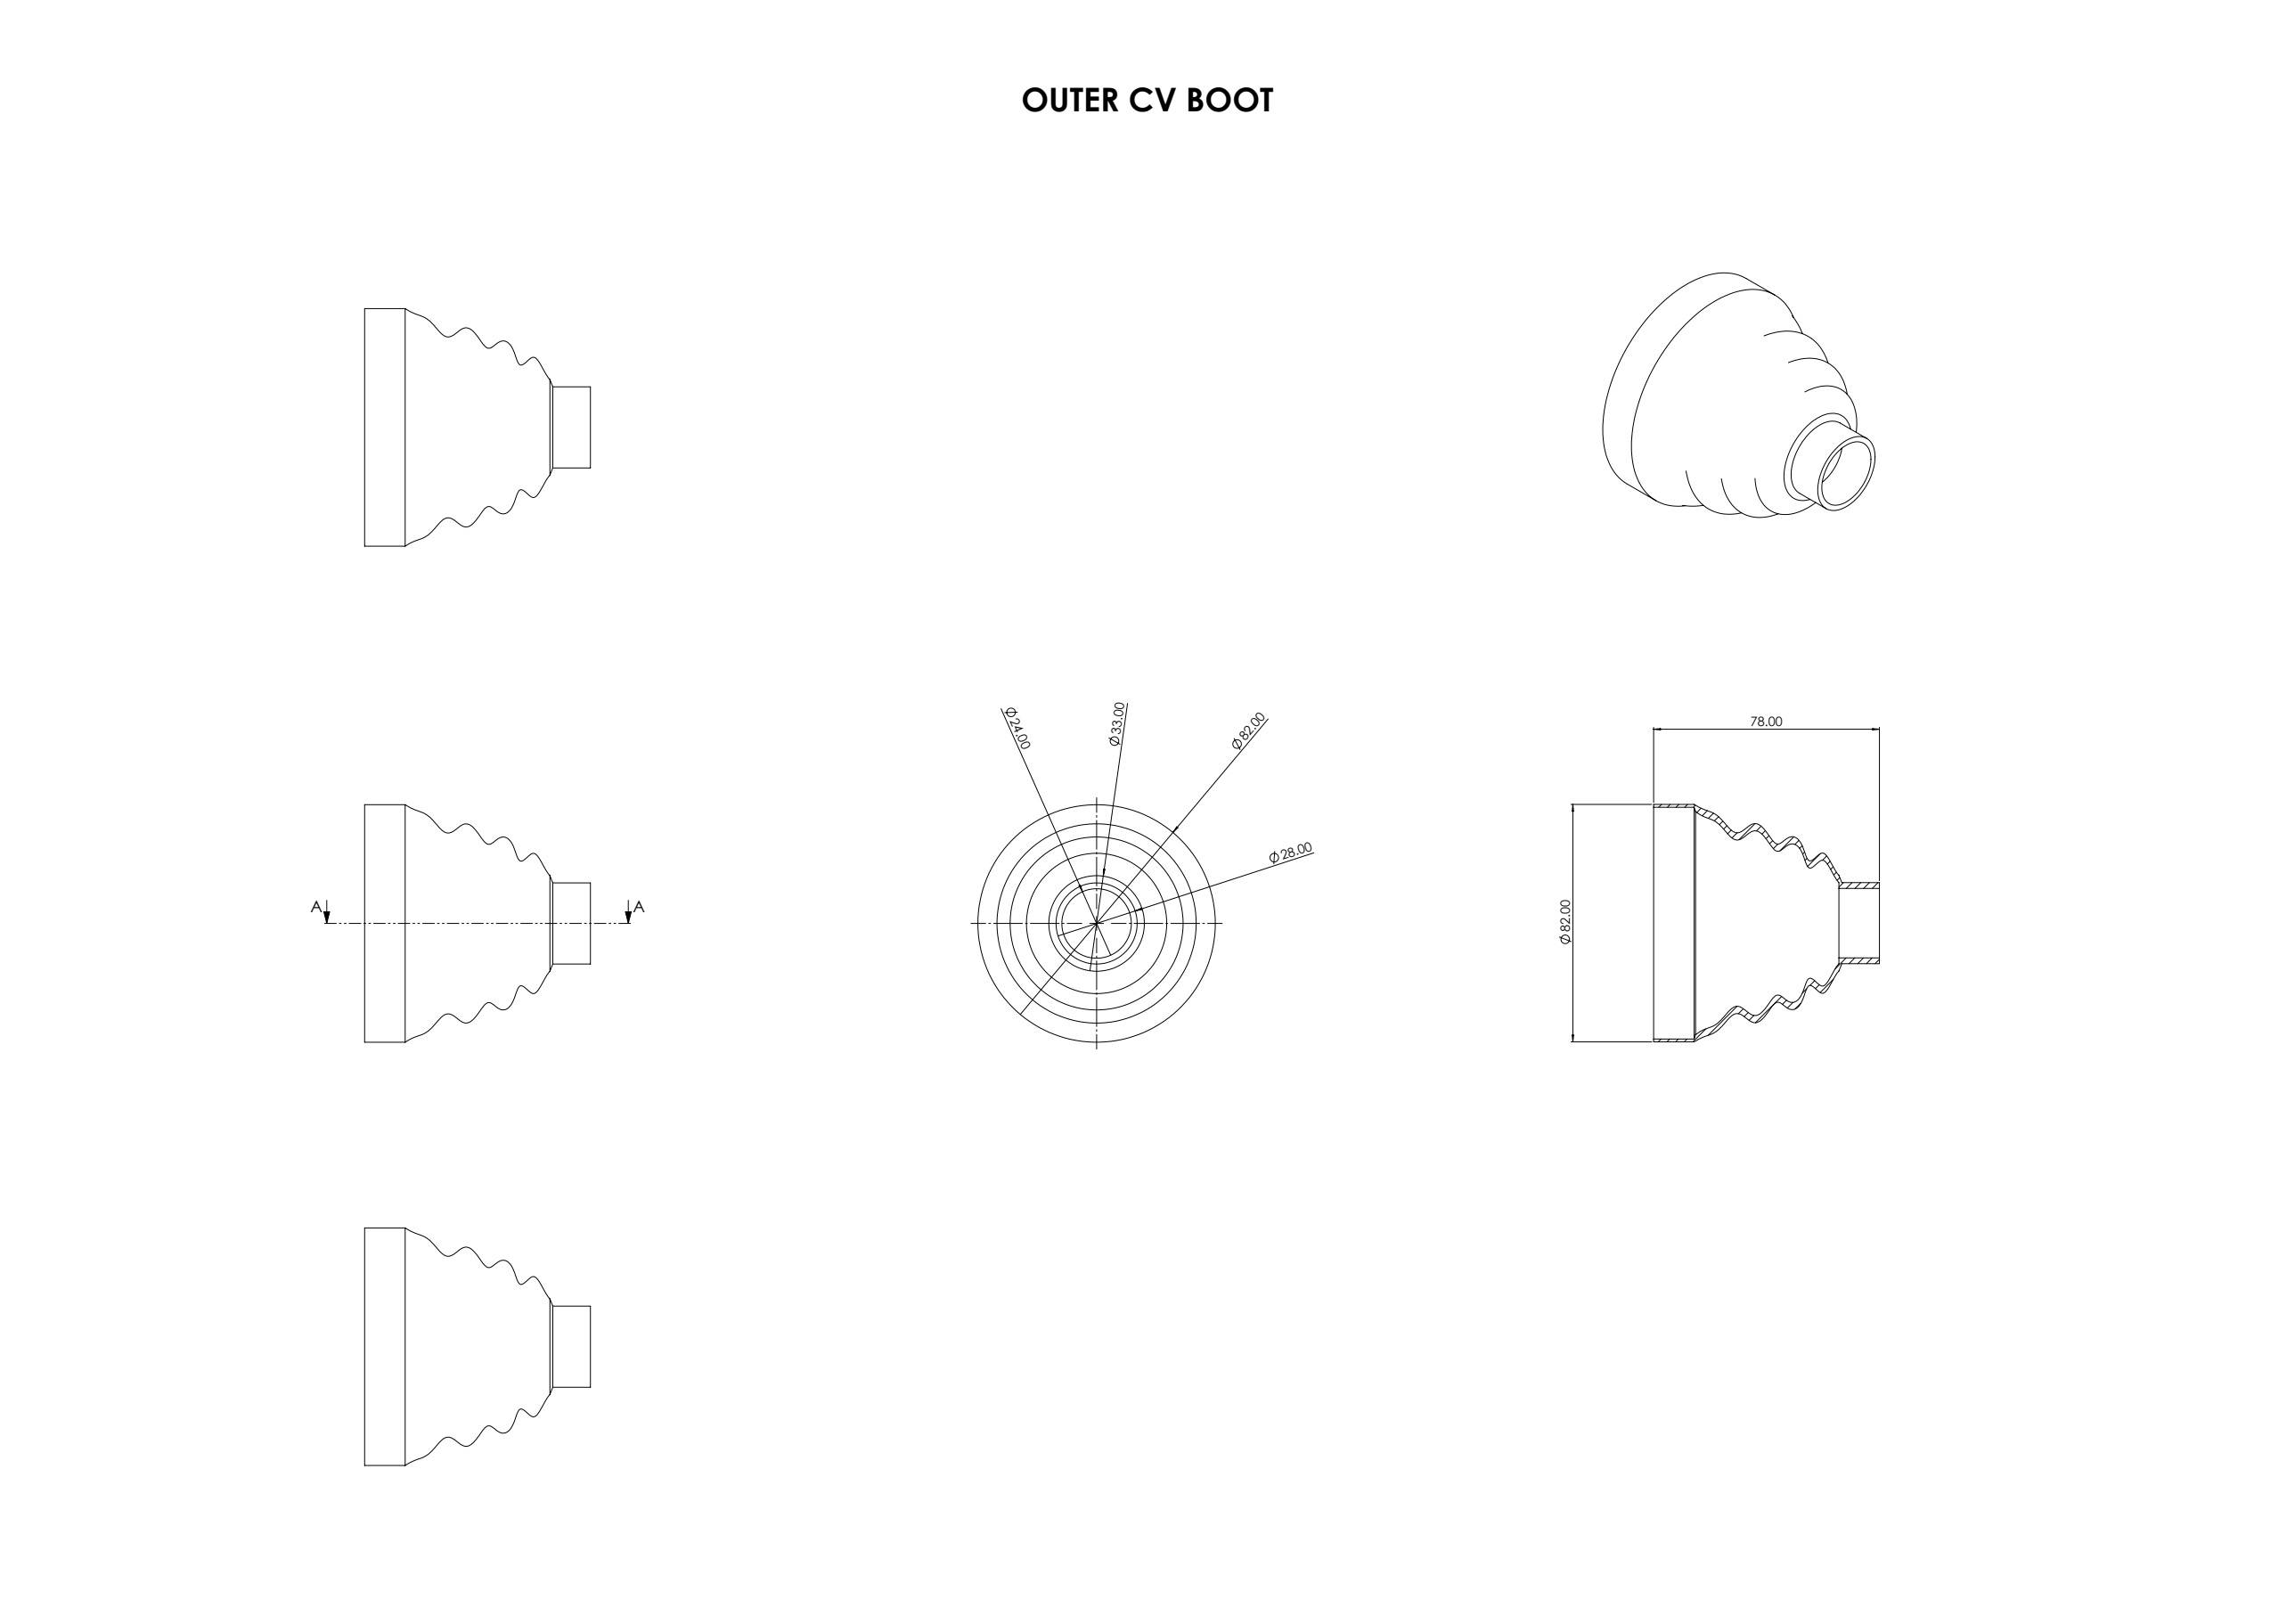
ISO-10303-21;
HEADER;
/* Generated by software containing ST-Developer
 * from STEP Tools, Inc. (www.steptools.com) 
 */

FILE_DESCRIPTION(
/* description */ (''),
/* implementation_level */ '2;1');

FILE_NAME(
/* name */ '07_Outer_CV_Boot.step',
/* time_stamp */ '2026-10-11T12:57:03-07:00',
/* author */ (''),
/* organization */ (''),
/* preprocessor_version */ 'ST-DEVELOPER v20.2',
/* originating_system */ 'Autodesk Translation Framework v15.15.0.0',
/* authorisation */ '');

FILE_SCHEMA (('AUTOMOTIVE_DESIGN { 1 0 10303 214 3 1 1 }'));
ENDSEC;

DATA;
#10=MECHANICAL_DESIGN_GEOMETRIC_PRESENTATION_REPRESENTATION('',(#262),#90374);
#228=SHAPE_REPRESENTATION_RELATIONSHIP('SRR','None',#90447,#245);
#245=ADVANCED_BREP_SHAPE_REPRESENTATION('',(#279),#90363);
#262=STYLED_ITEM('',(#90680),#279);
#279=MANIFOLD_SOLID_BREP('Body1',#40351);
#687=CONICAL_SURFACE('',#43806,15.25,1.19028994968254);
#688=CONICAL_SURFACE('',#43818,39.25,1.24904577239827);
#1066=FACE_BOUND('',#6231,.T.);
#1067=FACE_BOUND('',#6237,.T.);
#1068=FACE_BOUND('',#6240,.T.);
#1436=PLANE('',#43799);
#1437=PLANE('',#43810);
#1438=PLANE('',#43814);
#1831=(
BOUNDED_CURVE()
B_SPLINE_CURVE(5,(#82013,#82014,#82015,#82016,#82017,#82018,#82019,#82020,
#82021,#82022,#82023,#82024,#82025,#82026,#82027,#82028,#82029,#82030,#82031,
#82032,#82033,#82034,#82035,#82036,#82037,#82038,#82039,#82040,#82041,#82042,
#82043,#82044,#82045,#82046,#82047,#82048,#82049,#82050,#82051,#82052,#82053,
#82054,#82055,#82056,#82057,#82058,#82059,#82060,#82061,#82062,#82063,#82064,
#82065,#82066,#82067,#82068,#82069,#82070,#82071,#82072,#82073,#82074,#82075,
#82076,#82077,#82078,#82079,#82080,#82081,#82082,#82083,#82084,#82085,#82086,
#82087,#82088,#82089,#82090,#82091,#82092,#82093,#82094,#82095,#82096,#82097),
 .UNSPECIFIED.,.F.,.F.)
B_SPLINE_CURVE_WITH_KNOTS((6,1,1,1,1,1,1,1,1,1,1,1,1,1,1,1,1,1,1,1,1,1,
1,1,1,1,1,1,1,1,1,1,1,1,1,1,1,1,1,1,1,1,1,1,1,1,1,1,1,1,1,1,1,1,1,1,1,1,
1,1,1,1,1,1,1,1,1,1,1,1,1,1,1,1,1,1,1,1,1,1,6),(0.,0.0125,0.025,0.0375,
0.05,0.0625,0.075,0.0875,0.1,0.1125,0.125,0.1375,0.15,0.1625,0.175,0.1875,
0.2,0.2125,0.225,0.2375,0.25,0.2625,0.275,0.2875,0.3,0.3125,0.325,0.3375,
0.35,0.3625,0.375,0.3875,0.4,0.4125,0.425,0.4375,0.45,0.4625,0.475,0.4875,
0.5,0.5125,0.525,0.5375,0.55,0.5625,0.575,0.5875,0.6,0.6125,0.625,0.6375,
0.65,0.6625,0.675,0.6875,0.7,0.712499999999999,0.724999999999999,0.737499999999999,
0.749999999999999,0.762499999999999,0.774999999999999,0.787499999999999,
0.799999999999999,0.812499999999999,0.824999999999999,0.837499999999999,
0.849999999999999,0.862499999999999,0.874999999999999,0.887499999999999,
0.899999999999999,0.912499999999999,0.924999999999999,0.937499999999999,
0.949999999999999,0.962499999999999,0.974999999999999,0.987499999999998,
1.),.UNSPECIFIED.)
CURVE()
GEOMETRIC_REPRESENTATION_ITEM()
RATIONAL_B_SPLINE_CURVE((1.,1.,1.,1.,1.,1.,1.,1.,1.,1.,1.,1.,1.,1.,1.,1.,
1.,1.,1.,1.,1.,1.,1.,1.,1.,1.,1.,1.,1.,1.,1.,1.,1.,1.,1.,1.,1.,1.,1.,1.,
1.,1.,1.,1.,1.,1.,1.,1.,1.,1.,1.,1.,1.,1.,1.,1.,1.,1.,1.,1.,1.,1.,1.,1.,
1.,1.,1.,1.,1.,1.,1.,1.,1.,1.,1.,1.,1.,1.,1.,1.,1.,1.,1.,1.,1.))
REPRESENTATION_ITEM('')
);
#1832=(
BOUNDED_CURVE()
B_SPLINE_CURVE(5,(#82885,#82886,#82887,#82888,#82889,#82890,#82891,#82892,
#82893,#82894,#82895,#82896,#82897,#82898,#82899,#82900,#82901,#82902,#82903,
#82904,#82905,#82906,#82907,#82908,#82909,#82910,#82911,#82912,#82913,#82914,
#82915,#82916,#82917,#82918,#82919,#82920,#82921,#82922,#82923,#82924,#82925,
#82926,#82927,#82928,#82929,#82930,#82931,#82932,#82933,#82934,#82935,#82936,
#82937,#82938,#82939,#82940,#82941,#82942,#82943,#82944,#82945,#82946,#82947,
#82948,#82949,#82950,#82951,#82952,#82953,#82954,#82955,#82956,#82957,#82958,
#82959,#82960,#82961,#82962,#82963,#82964,#82965,#82966,#82967,#82968,#82969),
 .UNSPECIFIED.,.F.,.F.)
B_SPLINE_CURVE_WITH_KNOTS((6,1,1,1,1,1,1,1,1,1,1,1,1,1,1,1,1,1,1,1,1,1,
1,1,1,1,1,1,1,1,1,1,1,1,1,1,1,1,1,1,1,1,1,1,1,1,1,1,1,1,1,1,1,1,1,1,1,1,
1,1,1,1,1,1,1,1,1,1,1,1,1,1,1,1,1,1,1,1,1,1,6),(0.,0.0125,0.025,0.0375,
0.05,0.0625,0.075,0.0875,0.1,0.1125,0.125,0.1375,0.15,0.1625,0.175,0.1875,
0.2,0.2125,0.225,0.2375,0.25,0.2625,0.275,0.2875,0.3,0.3125,0.325,0.3375,
0.35,0.3625,0.375,0.3875,0.4,0.4125,0.425,0.4375,0.45,0.4625,0.475,0.4875,
0.5,0.5125,0.525,0.5375,0.55,0.5625,0.575,0.5875,0.6,0.6125,0.625,0.6375,
0.65,0.6625,0.675,0.6875,0.7,0.712499999999999,0.724999999999999,0.737499999999999,
0.749999999999999,0.762499999999999,0.774999999999999,0.787499999999999,
0.799999999999999,0.812499999999999,0.824999999999999,0.837499999999999,
0.849999999999999,0.862499999999999,0.874999999999999,0.887499999999999,
0.899999999999999,0.912499999999999,0.924999999999999,0.937499999999999,
0.949999999999999,0.962499999999999,0.974999999999999,0.987499999999998,
1.),.UNSPECIFIED.)
CURVE()
GEOMETRIC_REPRESENTATION_ITEM()
RATIONAL_B_SPLINE_CURVE((1.,1.,1.,1.,1.,1.,1.,1.,1.,1.,1.,1.,1.,1.,1.,1.,
1.,1.,1.,1.,1.,1.,1.,1.,1.,1.,1.,1.,1.,1.,1.,1.,1.,1.,1.,1.,1.,1.,1.,1.,
1.,1.,1.,1.,1.,1.,1.,1.,1.,1.,1.,1.,1.,1.,1.,1.,1.,1.,1.,1.,1.,1.,1.,1.,
1.,1.,1.,1.,1.,1.,1.,1.,1.,1.,1.,1.,1.,1.,1.,1.,1.,1.,1.,1.,1.))
REPRESENTATION_ITEM('')
);
#1934=(
BOUNDED_SURFACE()
B_SPLINE_SURFACE(5,2,((#81247,#81248,#81249,#81250,#81251,#81252,#81253,
#81254,#81255),(#81256,#81257,#81258,#81259,#81260,#81261,#81262,#81263,
#81264),(#81265,#81266,#81267,#81268,#81269,#81270,#81271,#81272,#81273),
(#81274,#81275,#81276,#81277,#81278,#81279,#81280,#81281,#81282),(#81283,
#81284,#81285,#81286,#81287,#81288,#81289,#81290,#81291),(#81292,#81293,
#81294,#81295,#81296,#81297,#81298,#81299,#81300),(#81301,#81302,#81303,
#81304,#81305,#81306,#81307,#81308,#81309),(#81310,#81311,#81312,#81313,
#81314,#81315,#81316,#81317,#81318),(#81319,#81320,#81321,#81322,#81323,
#81324,#81325,#81326,#81327),(#81328,#81329,#81330,#81331,#81332,#81333,
#81334,#81335,#81336),(#81337,#81338,#81339,#81340,#81341,#81342,#81343,
#81344,#81345),(#81346,#81347,#81348,#81349,#81350,#81351,#81352,#81353,
#81354),(#81355,#81356,#81357,#81358,#81359,#81360,#81361,#81362,#81363),
(#81364,#81365,#81366,#81367,#81368,#81369,#81370,#81371,#81372),(#81373,
#81374,#81375,#81376,#81377,#81378,#81379,#81380,#81381),(#81382,#81383,
#81384,#81385,#81386,#81387,#81388,#81389,#81390),(#81391,#81392,#81393,
#81394,#81395,#81396,#81397,#81398,#81399),(#81400,#81401,#81402,#81403,
#81404,#81405,#81406,#81407,#81408),(#81409,#81410,#81411,#81412,#81413,
#81414,#81415,#81416,#81417),(#81418,#81419,#81420,#81421,#81422,#81423,
#81424,#81425,#81426),(#81427,#81428,#81429,#81430,#81431,#81432,#81433,
#81434,#81435),(#81436,#81437,#81438,#81439,#81440,#81441,#81442,#81443,
#81444),(#81445,#81446,#81447,#81448,#81449,#81450,#81451,#81452,#81453),
(#81454,#81455,#81456,#81457,#81458,#81459,#81460,#81461,#81462),(#81463,
#81464,#81465,#81466,#81467,#81468,#81469,#81470,#81471),(#81472,#81473,
#81474,#81475,#81476,#81477,#81478,#81479,#81480),(#81481,#81482,#81483,
#81484,#81485,#81486,#81487,#81488,#81489),(#81490,#81491,#81492,#81493,
#81494,#81495,#81496,#81497,#81498),(#81499,#81500,#81501,#81502,#81503,
#81504,#81505,#81506,#81507),(#81508,#81509,#81510,#81511,#81512,#81513,
#81514,#81515,#81516),(#81517,#81518,#81519,#81520,#81521,#81522,#81523,
#81524,#81525),(#81526,#81527,#81528,#81529,#81530,#81531,#81532,#81533,
#81534),(#81535,#81536,#81537,#81538,#81539,#81540,#81541,#81542,#81543),
(#81544,#81545,#81546,#81547,#81548,#81549,#81550,#81551,#81552),(#81553,
#81554,#81555,#81556,#81557,#81558,#81559,#81560,#81561),(#81562,#81563,
#81564,#81565,#81566,#81567,#81568,#81569,#81570),(#81571,#81572,#81573,
#81574,#81575,#81576,#81577,#81578,#81579),(#81580,#81581,#81582,#81583,
#81584,#81585,#81586,#81587,#81588),(#81589,#81590,#81591,#81592,#81593,
#81594,#81595,#81596,#81597),(#81598,#81599,#81600,#81601,#81602,#81603,
#81604,#81605,#81606),(#81607,#81608,#81609,#81610,#81611,#81612,#81613,
#81614,#81615),(#81616,#81617,#81618,#81619,#81620,#81621,#81622,#81623,
#81624),(#81625,#81626,#81627,#81628,#81629,#81630,#81631,#81632,#81633),
(#81634,#81635,#81636,#81637,#81638,#81639,#81640,#81641,#81642),(#81643,
#81644,#81645,#81646,#81647,#81648,#81649,#81650,#81651),(#81652,#81653,
#81654,#81655,#81656,#81657,#81658,#81659,#81660),(#81661,#81662,#81663,
#81664,#81665,#81666,#81667,#81668,#81669),(#81670,#81671,#81672,#81673,
#81674,#81675,#81676,#81677,#81678),(#81679,#81680,#81681,#81682,#81683,
#81684,#81685,#81686,#81687),(#81688,#81689,#81690,#81691,#81692,#81693,
#81694,#81695,#81696),(#81697,#81698,#81699,#81700,#81701,#81702,#81703,
#81704,#81705),(#81706,#81707,#81708,#81709,#81710,#81711,#81712,#81713,
#81714),(#81715,#81716,#81717,#81718,#81719,#81720,#81721,#81722,#81723),
(#81724,#81725,#81726,#81727,#81728,#81729,#81730,#81731,#81732),(#81733,
#81734,#81735,#81736,#81737,#81738,#81739,#81740,#81741),(#81742,#81743,
#81744,#81745,#81746,#81747,#81748,#81749,#81750),(#81751,#81752,#81753,
#81754,#81755,#81756,#81757,#81758,#81759),(#81760,#81761,#81762,#81763,
#81764,#81765,#81766,#81767,#81768),(#81769,#81770,#81771,#81772,#81773,
#81774,#81775,#81776,#81777),(#81778,#81779,#81780,#81781,#81782,#81783,
#81784,#81785,#81786),(#81787,#81788,#81789,#81790,#81791,#81792,#81793,
#81794,#81795),(#81796,#81797,#81798,#81799,#81800,#81801,#81802,#81803,
#81804),(#81805,#81806,#81807,#81808,#81809,#81810,#81811,#81812,#81813),
(#81814,#81815,#81816,#81817,#81818,#81819,#81820,#81821,#81822),(#81823,
#81824,#81825,#81826,#81827,#81828,#81829,#81830,#81831),(#81832,#81833,
#81834,#81835,#81836,#81837,#81838,#81839,#81840),(#81841,#81842,#81843,
#81844,#81845,#81846,#81847,#81848,#81849),(#81850,#81851,#81852,#81853,
#81854,#81855,#81856,#81857,#81858),(#81859,#81860,#81861,#81862,#81863,
#81864,#81865,#81866,#81867),(#81868,#81869,#81870,#81871,#81872,#81873,
#81874,#81875,#81876),(#81877,#81878,#81879,#81880,#81881,#81882,#81883,
#81884,#81885),(#81886,#81887,#81888,#81889,#81890,#81891,#81892,#81893,
#81894),(#81895,#81896,#81897,#81898,#81899,#81900,#81901,#81902,#81903),
(#81904,#81905,#81906,#81907,#81908,#81909,#81910,#81911,#81912),(#81913,
#81914,#81915,#81916,#81917,#81918,#81919,#81920,#81921),(#81922,#81923,
#81924,#81925,#81926,#81927,#81928,#81929,#81930),(#81931,#81932,#81933,
#81934,#81935,#81936,#81937,#81938,#81939),(#81940,#81941,#81942,#81943,
#81944,#81945,#81946,#81947,#81948),(#81949,#81950,#81951,#81952,#81953,
#81954,#81955,#81956,#81957),(#81958,#81959,#81960,#81961,#81962,#81963,
#81964,#81965,#81966),(#81967,#81968,#81969,#81970,#81971,#81972,#81973,
#81974,#81975),(#81976,#81977,#81978,#81979,#81980,#81981,#81982,#81983,
#81984),(#81985,#81986,#81987,#81988,#81989,#81990,#81991,#81992,#81993),
(#81994,#81995,#81996,#81997,#81998,#81999,#82000,#82001,#82002),(#82003,
#82004,#82005,#82006,#82007,#82008,#82009,#82010,#82011)),.UNSPECIFIED.,
 .F.,.T.,.F.)
B_SPLINE_SURFACE_WITH_KNOTS((6,1,1,1,1,1,1,1,1,1,1,1,1,1,1,1,1,1,1,1,1,
1,1,1,1,1,1,1,1,1,1,1,1,1,1,1,1,1,1,1,1,1,1,1,1,1,1,1,1,1,1,1,1,1,1,1,1,
1,1,1,1,1,1,1,1,1,1,1,1,1,1,1,1,1,1,1,1,1,1,1,6),(3,2,2,2,3),(-1.,-0.987499999999998,
-0.974999999999999,-0.962499999999999,-0.949999999999999,-0.937499999999999,
-0.924999999999999,-0.912499999999999,-0.899999999999999,-0.887499999999999,
-0.874999999999999,-0.862499999999999,-0.849999999999999,-0.837499999999999,
-0.824999999999999,-0.812499999999999,-0.799999999999999,-0.787499999999999,
-0.774999999999999,-0.762499999999999,-0.749999999999999,-0.737499999999999,
-0.724999999999999,-0.712499999999999,-0.7,-0.6875,-0.675,-0.6625,-0.65,
-0.6375,-0.625,-0.6125,-0.6,-0.5875,-0.575,-0.5625,-0.55,-0.5375,-0.525,
-0.5125,-0.5,-0.4875,-0.475,-0.4625,-0.45,-0.4375,-0.425,-0.4125,-0.4,-0.3875,
-0.375,-0.3625,-0.35,-0.3375,-0.325,-0.3125,-0.3,-0.2875,-0.275,-0.2625,
-0.25,-0.2375,-0.225,-0.2125,-0.2,-0.1875,-0.175,-0.1625,-0.15,-0.1375,
-0.125,-0.1125,-0.1,-0.0875,-0.075,-0.0625,-0.05,-0.0375,-0.025,-0.0125,
0.),(0.,1.5707963267949,3.14159265358979,4.71238898038469,6.28318530717959),
 .UNSPECIFIED.)
GEOMETRIC_REPRESENTATION_ITEM()
RATIONAL_B_SPLINE_SURFACE(((1.,0.707106781186548,1.,0.707106781186548,1.,
0.707106781186548,1.,0.707106781186548,1.),(1.,0.707106781186548,1.,0.707106781186548,
1.,0.707106781186548,1.,0.707106781186548,1.),(1.,0.707106781186548,1.,
0.707106781186548,1.,0.707106781186548,1.,0.707106781186548,1.),(1.,0.707106781186548,
1.,0.707106781186548,1.,0.707106781186548,1.,0.707106781186548,1.),(1.,
0.707106781186548,1.,0.707106781186548,1.,0.707106781186548,1.,0.707106781186548,
1.),(1.,0.707106781186548,1.,0.707106781186548,1.,0.707106781186548,1.,
0.707106781186548,1.),(1.,0.707106781186548,1.,0.707106781186548,1.,0.707106781186548,
1.,0.707106781186548,1.),(1.,0.707106781186548,1.,0.707106781186548,1.,
0.707106781186548,1.,0.707106781186548,1.),(1.,0.707106781186548,1.,0.707106781186548,
1.,0.707106781186548,1.,0.707106781186548,1.),(1.,0.707106781186548,1.,
0.707106781186548,1.,0.707106781186548,1.,0.707106781186548,1.),(1.,0.707106781186548,
1.,0.707106781186548,1.,0.707106781186548,1.,0.707106781186548,1.),(1.,
0.707106781186548,1.,0.707106781186548,1.,0.707106781186548,1.,0.707106781186548,
1.),(1.,0.707106781186548,1.,0.707106781186548,1.,0.707106781186548,1.,
0.707106781186548,1.),(1.,0.707106781186548,1.,0.707106781186548,1.,0.707106781186548,
1.,0.707106781186548,1.),(1.,0.707106781186548,1.,0.707106781186548,1.,
0.707106781186548,1.,0.707106781186548,1.),(1.,0.707106781186548,1.,0.707106781186548,
1.,0.707106781186548,1.,0.707106781186548,1.),(1.,0.707106781186548,1.,
0.707106781186548,1.,0.707106781186548,1.,0.707106781186548,1.),(1.,0.707106781186548,
1.,0.707106781186548,1.,0.707106781186548,1.,0.707106781186548,1.),(1.,
0.707106781186548,1.,0.707106781186548,1.,0.707106781186548,1.,0.707106781186548,
1.),(1.,0.707106781186548,1.,0.707106781186548,1.,0.707106781186548,1.,
0.707106781186548,1.),(1.,0.707106781186548,1.,0.707106781186548,1.,0.707106781186548,
1.,0.707106781186548,1.),(1.,0.707106781186548,1.,0.707106781186548,1.,
0.707106781186548,1.,0.707106781186548,1.),(1.,0.707106781186548,1.,0.707106781186548,
1.,0.707106781186548,1.,0.707106781186548,1.),(1.,0.707106781186548,1.,
0.707106781186548,1.,0.707106781186548,1.,0.707106781186548,1.),(1.,0.707106781186548,
1.,0.707106781186548,1.,0.707106781186548,1.,0.707106781186548,1.),(1.,
0.707106781186548,1.,0.707106781186548,1.,0.707106781186548,1.,0.707106781186548,
1.),(1.,0.707106781186548,1.,0.707106781186548,1.,0.707106781186548,1.,
0.707106781186548,1.),(1.,0.707106781186548,1.,0.707106781186548,1.,0.707106781186548,
1.,0.707106781186548,1.),(1.,0.707106781186548,1.,0.707106781186548,1.,
0.707106781186548,1.,0.707106781186548,1.),(1.,0.707106781186548,1.,0.707106781186548,
1.,0.707106781186548,1.,0.707106781186548,1.),(1.,0.707106781186548,1.,
0.707106781186548,1.,0.707106781186548,1.,0.707106781186548,1.),(1.,0.707106781186548,
1.,0.707106781186548,1.,0.707106781186548,1.,0.707106781186548,1.),(1.,
0.707106781186548,1.,0.707106781186548,1.,0.707106781186548,1.,0.707106781186548,
1.),(1.,0.707106781186548,1.,0.707106781186548,1.,0.707106781186548,1.,
0.707106781186548,1.),(1.,0.707106781186548,1.,0.707106781186548,1.,0.707106781186548,
1.,0.707106781186548,1.),(1.,0.707106781186548,1.,0.707106781186548,1.,
0.707106781186548,1.,0.707106781186548,1.),(1.,0.707106781186548,1.,0.707106781186548,
1.,0.707106781186548,1.,0.707106781186548,1.),(1.,0.707106781186548,1.,
0.707106781186548,1.,0.707106781186548,1.,0.707106781186548,1.),(1.,0.707106781186548,
1.,0.707106781186548,1.,0.707106781186548,1.,0.707106781186548,1.),(1.,
0.707106781186548,1.,0.707106781186548,1.,0.707106781186548,1.,0.707106781186548,
1.),(1.,0.707106781186548,1.,0.707106781186548,1.,0.707106781186548,1.,
0.707106781186548,1.),(1.,0.707106781186548,1.,0.707106781186548,1.,0.707106781186548,
1.,0.707106781186548,1.),(1.,0.707106781186548,1.,0.707106781186548,1.,
0.707106781186548,1.,0.707106781186548,1.),(1.,0.707106781186548,1.,0.707106781186548,
1.,0.707106781186548,1.,0.707106781186548,1.),(1.,0.707106781186548,1.,
0.707106781186548,1.,0.707106781186548,1.,0.707106781186548,1.),(1.,0.707106781186548,
1.,0.707106781186548,1.,0.707106781186548,1.,0.707106781186548,1.),(1.,
0.707106781186548,1.,0.707106781186548,1.,0.707106781186548,1.,0.707106781186548,
1.),(1.,0.707106781186548,1.,0.707106781186548,1.,0.707106781186548,1.,
0.707106781186548,1.),(1.,0.707106781186548,1.,0.707106781186548,1.,0.707106781186548,
1.,0.707106781186548,1.),(1.,0.707106781186548,1.,0.707106781186548,1.,
0.707106781186548,1.,0.707106781186548,1.),(1.,0.707106781186548,1.,0.707106781186548,
1.,0.707106781186548,1.,0.707106781186548,1.),(1.,0.707106781186548,1.,
0.707106781186548,1.,0.707106781186548,1.,0.707106781186548,1.),(1.,0.707106781186548,
1.,0.707106781186548,1.,0.707106781186548,1.,0.707106781186548,1.),(1.,
0.707106781186548,1.,0.707106781186548,1.,0.707106781186548,1.,0.707106781186548,
1.),(1.,0.707106781186548,1.,0.707106781186548,1.,0.707106781186548,1.,
0.707106781186548,1.),(1.,0.707106781186548,1.,0.707106781186548,1.,0.707106781186548,
1.,0.707106781186548,1.),(1.,0.707106781186548,1.,0.707106781186548,1.,
0.707106781186548,1.,0.707106781186548,1.),(1.,0.707106781186548,1.,0.707106781186548,
1.,0.707106781186548,1.,0.707106781186548,1.),(1.,0.707106781186548,1.,
0.707106781186548,1.,0.707106781186548,1.,0.707106781186548,1.),(1.,0.707106781186548,
1.,0.707106781186548,1.,0.707106781186548,1.,0.707106781186548,1.),(1.,
0.707106781186548,1.,0.707106781186548,1.,0.707106781186548,1.,0.707106781186548,
1.),(1.,0.707106781186548,1.,0.707106781186548,1.,0.707106781186548,1.,
0.707106781186548,1.),(1.,0.707106781186548,1.,0.707106781186548,1.,0.707106781186548,
1.,0.707106781186548,1.),(1.,0.707106781186548,1.,0.707106781186548,1.,
0.707106781186548,1.,0.707106781186548,1.),(1.,0.707106781186548,1.,0.707106781186548,
1.,0.707106781186548,1.,0.707106781186548,1.),(1.,0.707106781186548,1.,
0.707106781186548,1.,0.707106781186548,1.,0.707106781186548,1.),(1.,0.707106781186548,
1.,0.707106781186548,1.,0.707106781186548,1.,0.707106781186548,1.),(1.,
0.707106781186548,1.,0.707106781186548,1.,0.707106781186548,1.,0.707106781186548,
1.),(1.,0.707106781186548,1.,0.707106781186548,1.,0.707106781186548,1.,
0.707106781186548,1.),(1.,0.707106781186548,1.,0.707106781186548,1.,0.707106781186548,
1.,0.707106781186548,1.),(1.,0.707106781186548,1.,0.707106781186548,1.,
0.707106781186548,1.,0.707106781186548,1.),(1.,0.707106781186548,1.,0.707106781186548,
1.,0.707106781186548,1.,0.707106781186548,1.),(1.,0.707106781186548,1.,
0.707106781186548,1.,0.707106781186548,1.,0.707106781186548,1.),(1.,0.707106781186548,
1.,0.707106781186548,1.,0.707106781186548,1.,0.707106781186548,1.),(1.,
0.707106781186548,1.,0.707106781186548,1.,0.707106781186548,1.,0.707106781186548,
1.),(1.,0.707106781186548,1.,0.707106781186548,1.,0.707106781186548,1.,
0.707106781186548,1.),(1.,0.707106781186548,1.,0.707106781186548,1.,0.707106781186548,
1.,0.707106781186548,1.),(1.,0.707106781186548,1.,0.707106781186548,1.,
0.707106781186548,1.,0.707106781186548,1.),(1.,0.707106781186548,1.,0.707106781186548,
1.,0.707106781186548,1.,0.707106781186548,1.),(1.,0.707106781186548,1.,
0.707106781186548,1.,0.707106781186548,1.,0.707106781186548,1.),(1.,0.707106781186548,
1.,0.707106781186548,1.,0.707106781186548,1.,0.707106781186548,1.),(1.,
0.707106781186548,1.,0.707106781186548,1.,0.707106781186548,1.,0.707106781186548,
1.),(1.,0.707106781186548,1.,0.707106781186548,1.,0.707106781186548,1.,
0.707106781186548,1.),(1.,0.707106781186548,1.,0.707106781186548,1.,0.707106781186548,
1.,0.707106781186548,1.),(1.,0.707106781186548,1.,0.707106781186548,1.,
0.707106781186548,1.,0.707106781186548,1.)))
REPRESENTATION_ITEM('')
SURFACE()
);
#1935=(
BOUNDED_SURFACE()
B_SPLINE_SURFACE(5,2,((#82119,#82120,#82121,#82122,#82123,#82124,#82125,
#82126,#82127),(#82128,#82129,#82130,#82131,#82132,#82133,#82134,#82135,
#82136),(#82137,#82138,#82139,#82140,#82141,#82142,#82143,#82144,#82145),
(#82146,#82147,#82148,#82149,#82150,#82151,#82152,#82153,#82154),(#82155,
#82156,#82157,#82158,#82159,#82160,#82161,#82162,#82163),(#82164,#82165,
#82166,#82167,#82168,#82169,#82170,#82171,#82172),(#82173,#82174,#82175,
#82176,#82177,#82178,#82179,#82180,#82181),(#82182,#82183,#82184,#82185,
#82186,#82187,#82188,#82189,#82190),(#82191,#82192,#82193,#82194,#82195,
#82196,#82197,#82198,#82199),(#82200,#82201,#82202,#82203,#82204,#82205,
#82206,#82207,#82208),(#82209,#82210,#82211,#82212,#82213,#82214,#82215,
#82216,#82217),(#82218,#82219,#82220,#82221,#82222,#82223,#82224,#82225,
#82226),(#82227,#82228,#82229,#82230,#82231,#82232,#82233,#82234,#82235),
(#82236,#82237,#82238,#82239,#82240,#82241,#82242,#82243,#82244),(#82245,
#82246,#82247,#82248,#82249,#82250,#82251,#82252,#82253),(#82254,#82255,
#82256,#82257,#82258,#82259,#82260,#82261,#82262),(#82263,#82264,#82265,
#82266,#82267,#82268,#82269,#82270,#82271),(#82272,#82273,#82274,#82275,
#82276,#82277,#82278,#82279,#82280),(#82281,#82282,#82283,#82284,#82285,
#82286,#82287,#82288,#82289),(#82290,#82291,#82292,#82293,#82294,#82295,
#82296,#82297,#82298),(#82299,#82300,#82301,#82302,#82303,#82304,#82305,
#82306,#82307),(#82308,#82309,#82310,#82311,#82312,#82313,#82314,#82315,
#82316),(#82317,#82318,#82319,#82320,#82321,#82322,#82323,#82324,#82325),
(#82326,#82327,#82328,#82329,#82330,#82331,#82332,#82333,#82334),(#82335,
#82336,#82337,#82338,#82339,#82340,#82341,#82342,#82343),(#82344,#82345,
#82346,#82347,#82348,#82349,#82350,#82351,#82352),(#82353,#82354,#82355,
#82356,#82357,#82358,#82359,#82360,#82361),(#82362,#82363,#82364,#82365,
#82366,#82367,#82368,#82369,#82370),(#82371,#82372,#82373,#82374,#82375,
#82376,#82377,#82378,#82379),(#82380,#82381,#82382,#82383,#82384,#82385,
#82386,#82387,#82388),(#82389,#82390,#82391,#82392,#82393,#82394,#82395,
#82396,#82397),(#82398,#82399,#82400,#82401,#82402,#82403,#82404,#82405,
#82406),(#82407,#82408,#82409,#82410,#82411,#82412,#82413,#82414,#82415),
(#82416,#82417,#82418,#82419,#82420,#82421,#82422,#82423,#82424),(#82425,
#82426,#82427,#82428,#82429,#82430,#82431,#82432,#82433),(#82434,#82435,
#82436,#82437,#82438,#82439,#82440,#82441,#82442),(#82443,#82444,#82445,
#82446,#82447,#82448,#82449,#82450,#82451),(#82452,#82453,#82454,#82455,
#82456,#82457,#82458,#82459,#82460),(#82461,#82462,#82463,#82464,#82465,
#82466,#82467,#82468,#82469),(#82470,#82471,#82472,#82473,#82474,#82475,
#82476,#82477,#82478),(#82479,#82480,#82481,#82482,#82483,#82484,#82485,
#82486,#82487),(#82488,#82489,#82490,#82491,#82492,#82493,#82494,#82495,
#82496),(#82497,#82498,#82499,#82500,#82501,#82502,#82503,#82504,#82505),
(#82506,#82507,#82508,#82509,#82510,#82511,#82512,#82513,#82514),(#82515,
#82516,#82517,#82518,#82519,#82520,#82521,#82522,#82523),(#82524,#82525,
#82526,#82527,#82528,#82529,#82530,#82531,#82532),(#82533,#82534,#82535,
#82536,#82537,#82538,#82539,#82540,#82541),(#82542,#82543,#82544,#82545,
#82546,#82547,#82548,#82549,#82550),(#82551,#82552,#82553,#82554,#82555,
#82556,#82557,#82558,#82559),(#82560,#82561,#82562,#82563,#82564,#82565,
#82566,#82567,#82568),(#82569,#82570,#82571,#82572,#82573,#82574,#82575,
#82576,#82577),(#82578,#82579,#82580,#82581,#82582,#82583,#82584,#82585,
#82586),(#82587,#82588,#82589,#82590,#82591,#82592,#82593,#82594,#82595),
(#82596,#82597,#82598,#82599,#82600,#82601,#82602,#82603,#82604),(#82605,
#82606,#82607,#82608,#82609,#82610,#82611,#82612,#82613),(#82614,#82615,
#82616,#82617,#82618,#82619,#82620,#82621,#82622),(#82623,#82624,#82625,
#82626,#82627,#82628,#82629,#82630,#82631),(#82632,#82633,#82634,#82635,
#82636,#82637,#82638,#82639,#82640),(#82641,#82642,#82643,#82644,#82645,
#82646,#82647,#82648,#82649),(#82650,#82651,#82652,#82653,#82654,#82655,
#82656,#82657,#82658),(#82659,#82660,#82661,#82662,#82663,#82664,#82665,
#82666,#82667),(#82668,#82669,#82670,#82671,#82672,#82673,#82674,#82675,
#82676),(#82677,#82678,#82679,#82680,#82681,#82682,#82683,#82684,#82685),
(#82686,#82687,#82688,#82689,#82690,#82691,#82692,#82693,#82694),(#82695,
#82696,#82697,#82698,#82699,#82700,#82701,#82702,#82703),(#82704,#82705,
#82706,#82707,#82708,#82709,#82710,#82711,#82712),(#82713,#82714,#82715,
#82716,#82717,#82718,#82719,#82720,#82721),(#82722,#82723,#82724,#82725,
#82726,#82727,#82728,#82729,#82730),(#82731,#82732,#82733,#82734,#82735,
#82736,#82737,#82738,#82739),(#82740,#82741,#82742,#82743,#82744,#82745,
#82746,#82747,#82748),(#82749,#82750,#82751,#82752,#82753,#82754,#82755,
#82756,#82757),(#82758,#82759,#82760,#82761,#82762,#82763,#82764,#82765,
#82766),(#82767,#82768,#82769,#82770,#82771,#82772,#82773,#82774,#82775),
(#82776,#82777,#82778,#82779,#82780,#82781,#82782,#82783,#82784),(#82785,
#82786,#82787,#82788,#82789,#82790,#82791,#82792,#82793),(#82794,#82795,
#82796,#82797,#82798,#82799,#82800,#82801,#82802),(#82803,#82804,#82805,
#82806,#82807,#82808,#82809,#82810,#82811),(#82812,#82813,#82814,#82815,
#82816,#82817,#82818,#82819,#82820),(#82821,#82822,#82823,#82824,#82825,
#82826,#82827,#82828,#82829),(#82830,#82831,#82832,#82833,#82834,#82835,
#82836,#82837,#82838),(#82839,#82840,#82841,#82842,#82843,#82844,#82845,
#82846,#82847),(#82848,#82849,#82850,#82851,#82852,#82853,#82854,#82855,
#82856),(#82857,#82858,#82859,#82860,#82861,#82862,#82863,#82864,#82865),
(#82866,#82867,#82868,#82869,#82870,#82871,#82872,#82873,#82874),(#82875,
#82876,#82877,#82878,#82879,#82880,#82881,#82882,#82883)),.UNSPECIFIED.,
 .F.,.T.,.F.)
B_SPLINE_SURFACE_WITH_KNOTS((6,1,1,1,1,1,1,1,1,1,1,1,1,1,1,1,1,1,1,1,1,
1,1,1,1,1,1,1,1,1,1,1,1,1,1,1,1,1,1,1,1,1,1,1,1,1,1,1,1,1,1,1,1,1,1,1,1,
1,1,1,1,1,1,1,1,1,1,1,1,1,1,1,1,1,1,1,1,1,1,1,6),(3,2,2,2,3),(-1.,-0.987499999999998,
-0.974999999999999,-0.962499999999999,-0.949999999999999,-0.937499999999999,
-0.924999999999999,-0.912499999999999,-0.899999999999999,-0.887499999999999,
-0.874999999999999,-0.862499999999999,-0.849999999999999,-0.837499999999999,
-0.824999999999999,-0.812499999999999,-0.799999999999999,-0.787499999999999,
-0.774999999999999,-0.762499999999999,-0.749999999999999,-0.737499999999999,
-0.724999999999999,-0.712499999999999,-0.7,-0.6875,-0.675,-0.6625,-0.65,
-0.6375,-0.625,-0.6125,-0.6,-0.5875,-0.575,-0.5625,-0.55,-0.5375,-0.525,
-0.5125,-0.5,-0.4875,-0.475,-0.4625,-0.45,-0.4375,-0.425,-0.4125,-0.4,-0.3875,
-0.375,-0.3625,-0.35,-0.3375,-0.325,-0.3125,-0.3,-0.2875,-0.275,-0.2625,
-0.25,-0.2375,-0.225,-0.2125,-0.2,-0.1875,-0.175,-0.1625,-0.15,-0.1375,
-0.125,-0.1125,-0.1,-0.0875,-0.075,-0.0625,-0.05,-0.0375,-0.025,-0.0125,
0.),(0.,1.5707963267949,3.14159265358979,4.71238898038469,6.28318530717959),
 .UNSPECIFIED.)
GEOMETRIC_REPRESENTATION_ITEM()
RATIONAL_B_SPLINE_SURFACE(((1.,0.707106781186548,1.,0.707106781186548,1.,
0.707106781186548,1.,0.707106781186548,1.),(1.,0.707106781186548,1.,0.707106781186548,
1.,0.707106781186548,1.,0.707106781186548,1.),(1.,0.707106781186548,1.,
0.707106781186548,1.,0.707106781186548,1.,0.707106781186548,1.),(1.,0.707106781186548,
1.,0.707106781186548,1.,0.707106781186548,1.,0.707106781186548,1.),(1.,
0.707106781186548,1.,0.707106781186548,1.,0.707106781186548,1.,0.707106781186548,
1.),(1.,0.707106781186548,1.,0.707106781186548,1.,0.707106781186548,1.,
0.707106781186548,1.),(1.,0.707106781186548,1.,0.707106781186548,1.,0.707106781186548,
1.,0.707106781186548,1.),(1.,0.707106781186548,1.,0.707106781186548,1.,
0.707106781186548,1.,0.707106781186548,1.),(1.,0.707106781186548,1.,0.707106781186548,
1.,0.707106781186548,1.,0.707106781186548,1.),(1.,0.707106781186548,1.,
0.707106781186548,1.,0.707106781186548,1.,0.707106781186548,1.),(1.,0.707106781186548,
1.,0.707106781186548,1.,0.707106781186548,1.,0.707106781186548,1.),(1.,
0.707106781186548,1.,0.707106781186548,1.,0.707106781186548,1.,0.707106781186548,
1.),(1.,0.707106781186548,1.,0.707106781186548,1.,0.707106781186548,1.,
0.707106781186548,1.),(1.,0.707106781186548,1.,0.707106781186548,1.,0.707106781186548,
1.,0.707106781186548,1.),(1.,0.707106781186548,1.,0.707106781186548,1.,
0.707106781186548,1.,0.707106781186548,1.),(1.,0.707106781186548,1.,0.707106781186548,
1.,0.707106781186548,1.,0.707106781186548,1.),(1.,0.707106781186548,1.,
0.707106781186548,1.,0.707106781186548,1.,0.707106781186548,1.),(1.,0.707106781186548,
1.,0.707106781186548,1.,0.707106781186548,1.,0.707106781186548,1.),(1.,
0.707106781186548,1.,0.707106781186548,1.,0.707106781186548,1.,0.707106781186548,
1.),(1.,0.707106781186548,1.,0.707106781186548,1.,0.707106781186548,1.,
0.707106781186548,1.),(1.,0.707106781186548,1.,0.707106781186548,1.,0.707106781186548,
1.,0.707106781186548,1.),(1.,0.707106781186548,1.,0.707106781186548,1.,
0.707106781186548,1.,0.707106781186548,1.),(1.,0.707106781186548,1.,0.707106781186548,
1.,0.707106781186548,1.,0.707106781186548,1.),(1.,0.707106781186548,1.,
0.707106781186548,1.,0.707106781186548,1.,0.707106781186548,1.),(1.,0.707106781186548,
1.,0.707106781186548,1.,0.707106781186548,1.,0.707106781186548,1.),(1.,
0.707106781186548,1.,0.707106781186548,1.,0.707106781186548,1.,0.707106781186548,
1.),(1.,0.707106781186548,1.,0.707106781186548,1.,0.707106781186548,1.,
0.707106781186548,1.),(1.,0.707106781186548,1.,0.707106781186548,1.,0.707106781186548,
1.,0.707106781186548,1.),(1.,0.707106781186548,1.,0.707106781186548,1.,
0.707106781186548,1.,0.707106781186548,1.),(1.,0.707106781186548,1.,0.707106781186548,
1.,0.707106781186548,1.,0.707106781186548,1.),(1.,0.707106781186548,1.,
0.707106781186548,1.,0.707106781186548,1.,0.707106781186548,1.),(1.,0.707106781186548,
1.,0.707106781186548,1.,0.707106781186548,1.,0.707106781186548,1.),(1.,
0.707106781186548,1.,0.707106781186548,1.,0.707106781186548,1.,0.707106781186548,
1.),(1.,0.707106781186548,1.,0.707106781186548,1.,0.707106781186548,1.,
0.707106781186548,1.),(1.,0.707106781186548,1.,0.707106781186548,1.,0.707106781186548,
1.,0.707106781186548,1.),(1.,0.707106781186548,1.,0.707106781186548,1.,
0.707106781186548,1.,0.707106781186548,1.),(1.,0.707106781186548,1.,0.707106781186548,
1.,0.707106781186548,1.,0.707106781186548,1.),(1.,0.707106781186548,1.,
0.707106781186548,1.,0.707106781186548,1.,0.707106781186548,1.),(1.,0.707106781186548,
1.,0.707106781186548,1.,0.707106781186548,1.,0.707106781186548,1.),(1.,
0.707106781186548,1.,0.707106781186548,1.,0.707106781186548,1.,0.707106781186548,
1.),(1.,0.707106781186548,1.,0.707106781186548,1.,0.707106781186548,1.,
0.707106781186548,1.),(1.,0.707106781186548,1.,0.707106781186548,1.,0.707106781186548,
1.,0.707106781186548,1.),(1.,0.707106781186548,1.,0.707106781186548,1.,
0.707106781186548,1.,0.707106781186548,1.),(1.,0.707106781186548,1.,0.707106781186548,
1.,0.707106781186548,1.,0.707106781186548,1.),(1.,0.707106781186548,1.,
0.707106781186548,1.,0.707106781186548,1.,0.707106781186548,1.),(1.,0.707106781186548,
1.,0.707106781186548,1.,0.707106781186548,1.,0.707106781186548,1.),(1.,
0.707106781186548,1.,0.707106781186548,1.,0.707106781186548,1.,0.707106781186548,
1.),(1.,0.707106781186548,1.,0.707106781186548,1.,0.707106781186548,1.,
0.707106781186548,1.),(1.,0.707106781186548,1.,0.707106781186548,1.,0.707106781186548,
1.,0.707106781186548,1.),(1.,0.707106781186548,1.,0.707106781186548,1.,
0.707106781186548,1.,0.707106781186548,1.),(1.,0.707106781186548,1.,0.707106781186548,
1.,0.707106781186548,1.,0.707106781186548,1.),(1.,0.707106781186548,1.,
0.707106781186548,1.,0.707106781186548,1.,0.707106781186548,1.),(1.,0.707106781186548,
1.,0.707106781186548,1.,0.707106781186548,1.,0.707106781186548,1.),(1.,
0.707106781186548,1.,0.707106781186548,1.,0.707106781186548,1.,0.707106781186548,
1.),(1.,0.707106781186548,1.,0.707106781186548,1.,0.707106781186548,1.,
0.707106781186548,1.),(1.,0.707106781186548,1.,0.707106781186548,1.,0.707106781186548,
1.,0.707106781186548,1.),(1.,0.707106781186548,1.,0.707106781186548,1.,
0.707106781186548,1.,0.707106781186548,1.),(1.,0.707106781186548,1.,0.707106781186548,
1.,0.707106781186548,1.,0.707106781186548,1.),(1.,0.707106781186548,1.,
0.707106781186548,1.,0.707106781186548,1.,0.707106781186548,1.),(1.,0.707106781186548,
1.,0.707106781186548,1.,0.707106781186548,1.,0.707106781186548,1.),(1.,
0.707106781186548,1.,0.707106781186548,1.,0.707106781186548,1.,0.707106781186548,
1.),(1.,0.707106781186548,1.,0.707106781186548,1.,0.707106781186548,1.,
0.707106781186548,1.),(1.,0.707106781186548,1.,0.707106781186548,1.,0.707106781186548,
1.,0.707106781186548,1.),(1.,0.707106781186548,1.,0.707106781186548,1.,
0.707106781186548,1.,0.707106781186548,1.),(1.,0.707106781186548,1.,0.707106781186548,
1.,0.707106781186548,1.,0.707106781186548,1.),(1.,0.707106781186548,1.,
0.707106781186548,1.,0.707106781186548,1.,0.707106781186548,1.),(1.,0.707106781186548,
1.,0.707106781186548,1.,0.707106781186548,1.,0.707106781186548,1.),(1.,
0.707106781186548,1.,0.707106781186548,1.,0.707106781186548,1.,0.707106781186548,
1.),(1.,0.707106781186548,1.,0.707106781186548,1.,0.707106781186548,1.,
0.707106781186548,1.),(1.,0.707106781186548,1.,0.707106781186548,1.,0.707106781186548,
1.,0.707106781186548,1.),(1.,0.707106781186548,1.,0.707106781186548,1.,
0.707106781186548,1.,0.707106781186548,1.),(1.,0.707106781186548,1.,0.707106781186548,
1.,0.707106781186548,1.,0.707106781186548,1.),(1.,0.707106781186548,1.,
0.707106781186548,1.,0.707106781186548,1.,0.707106781186548,1.),(1.,0.707106781186548,
1.,0.707106781186548,1.,0.707106781186548,1.,0.707106781186548,1.),(1.,
0.707106781186548,1.,0.707106781186548,1.,0.707106781186548,1.,0.707106781186548,
1.),(1.,0.707106781186548,1.,0.707106781186548,1.,0.707106781186548,1.,
0.707106781186548,1.),(1.,0.707106781186548,1.,0.707106781186548,1.,0.707106781186548,
1.,0.707106781186548,1.),(1.,0.707106781186548,1.,0.707106781186548,1.,
0.707106781186548,1.,0.707106781186548,1.),(1.,0.707106781186548,1.,0.707106781186548,
1.,0.707106781186548,1.,0.707106781186548,1.),(1.,0.707106781186548,1.,
0.707106781186548,1.,0.707106781186548,1.,0.707106781186548,1.),(1.,0.707106781186548,
1.,0.707106781186548,1.,0.707106781186548,1.,0.707106781186548,1.),(1.,
0.707106781186548,1.,0.707106781186548,1.,0.707106781186548,1.,0.707106781186548,
1.),(1.,0.707106781186548,1.,0.707106781186548,1.,0.707106781186548,1.,
0.707106781186548,1.),(1.,0.707106781186548,1.,0.707106781186548,1.,0.707106781186548,
1.,0.707106781186548,1.),(1.,0.707106781186548,1.,0.707106781186548,1.,
0.707106781186548,1.,0.707106781186548,1.)))
REPRESENTATION_ITEM('')
SURFACE()
);
#3806=FACE_OUTER_BOUND('',#6229,.T.);
#3807=FACE_OUTER_BOUND('',#6230,.T.);
#3808=FACE_OUTER_BOUND('',#6232,.T.);
#3809=FACE_OUTER_BOUND('',#6233,.T.);
#3810=FACE_OUTER_BOUND('',#6234,.T.);
#3811=FACE_OUTER_BOUND('',#6235,.T.);
#3812=FACE_OUTER_BOUND('',#6236,.T.);
#3813=FACE_OUTER_BOUND('',#6238,.T.);
#3814=FACE_OUTER_BOUND('',#6239,.T.);
#3815=FACE_OUTER_BOUND('',#6241,.T.);
#3816=FACE_OUTER_BOUND('',#6242,.T.);
#6229=EDGE_LOOP('',(#33267,#33268,#33269,#33270));
#6230=EDGE_LOOP('',(#33271));
#6231=EDGE_LOOP('',(#33272));
#6232=EDGE_LOOP('',(#33273,#33274,#33275,#33276,#33277));
#6233=EDGE_LOOP('',(#33278,#33279,#33280,#33281,#33282,#33283));
#6234=EDGE_LOOP('',(#33284,#33285,#33286,#33287,#33288));
#6235=EDGE_LOOP('',(#33289,#33290,#33291,#33292));
#6236=EDGE_LOOP('',(#33293));
#6237=EDGE_LOOP('',(#33294));
#6238=EDGE_LOOP('',(#33295,#33296,#33297,#33298));
#6239=EDGE_LOOP('',(#33299));
#6240=EDGE_LOOP('',(#33300));
#6241=EDGE_LOOP('',(#33301,#33302,#33303,#33304,#33305));
#6242=EDGE_LOOP('',(#33306,#33307,#33308,#33309,#33310));
#8679=CIRCLE('',#43797,40.);
#8680=CIRCLE('',#43798,40.);
#8681=CIRCLE('',#43800,41.);
#8682=CIRCLE('',#43802,41.);
#8683=CIRCLE('',#43803,41.);
#8684=CIRCLE('',#43804,16.5);
#8685=CIRCLE('',#43805,16.5);
#8686=CIRCLE('',#43807,14.);
#8687=CIRCLE('',#43809,14.);
#8688=CIRCLE('',#43811,12.);
#8689=CIRCLE('',#43813,12.);
#8690=CIRCLE('',#43815,14.);
#8691=CIRCLE('',#43816,38.5);
#8692=CIRCLE('',#43817,38.5);
#11841=LINE('',#81236,#14335);
#11842=LINE('',#81246,#14336);
#11843=LINE('',#82104,#14337);
#11844=LINE('',#82108,#14338);
#11845=LINE('',#82114,#14339);
#11846=LINE('',#82974,#14340);
#14335=VECTOR('',#53275,40.);
#14336=VECTOR('',#53288,41.);
#14337=VECTOR('',#53297,15.25);
#14338=VECTOR('',#53302,14.);
#14339=VECTOR('',#53309,12.);
#14340=VECTOR('',#53322,39.25);
#17774=VERTEX_POINT('',#81233);
#17775=VERTEX_POINT('',#81235);
#17776=VERTEX_POINT('',#81239);
#17777=VERTEX_POINT('',#81242);
#17778=VERTEX_POINT('',#81243);
#17779=VERTEX_POINT('',#82012);
#17780=VERTEX_POINT('',#82098);
#17781=VERTEX_POINT('',#82102);
#17782=VERTEX_POINT('',#82106);
#17783=VERTEX_POINT('',#82110);
#17784=VERTEX_POINT('',#82113);
#17785=VERTEX_POINT('',#82117);
#17786=VERTEX_POINT('',#82884);
#17787=VERTEX_POINT('',#82970);
#23145=EDGE_CURVE('',#17774,#17774,#8679,.T.);
#23146=EDGE_CURVE('',#17774,#17775,#11841,.T.);
#23147=EDGE_CURVE('',#17775,#17775,#8680,.T.);
#23148=EDGE_CURVE('',#17776,#17776,#8681,.T.);
#23149=EDGE_CURVE('',#17777,#17778,#8682,.T.);
#23150=EDGE_CURVE('',#17778,#17777,#8683,.T.);
#23151=EDGE_CURVE('',#17778,#17776,#11842,.T.);
#23152=EDGE_CURVE('',#17777,#17779,#1831,.T.);
#23153=EDGE_CURVE('',#17780,#17779,#8684,.T.);
#23154=EDGE_CURVE('',#17779,#17780,#8685,.T.);
#23155=EDGE_CURVE('',#17781,#17781,#8686,.T.);
#23156=EDGE_CURVE('',#17781,#17780,#11843,.T.);
#23157=EDGE_CURVE('',#17782,#17782,#8687,.T.);
#23158=EDGE_CURVE('',#17782,#17781,#11844,.T.);
#23159=EDGE_CURVE('',#17783,#17783,#8688,.T.);
#23160=EDGE_CURVE('',#17783,#17784,#11845,.T.);
#23161=EDGE_CURVE('',#17784,#17784,#8689,.T.);
#23162=EDGE_CURVE('',#17785,#17785,#8690,.T.);
#23163=EDGE_CURVE('',#17785,#17786,#1832,.T.);
#23164=EDGE_CURVE('',#17787,#17786,#8691,.T.);
#23165=EDGE_CURVE('',#17786,#17787,#8692,.T.);
#23166=EDGE_CURVE('',#17787,#17774,#11846,.T.);
#33267=ORIENTED_EDGE('',*,*,#23145,.T.);
#33268=ORIENTED_EDGE('',*,*,#23146,.T.);
#33269=ORIENTED_EDGE('',*,*,#23147,.F.);
#33270=ORIENTED_EDGE('',*,*,#23146,.F.);
#33271=ORIENTED_EDGE('',*,*,#23148,.F.);
#33272=ORIENTED_EDGE('',*,*,#23147,.T.);
#33273=ORIENTED_EDGE('',*,*,#23149,.F.);
#33274=ORIENTED_EDGE('',*,*,#23150,.F.);
#33275=ORIENTED_EDGE('',*,*,#23151,.T.);
#33276=ORIENTED_EDGE('',*,*,#23148,.T.);
#33277=ORIENTED_EDGE('',*,*,#23151,.F.);
#33278=ORIENTED_EDGE('',*,*,#23152,.F.);
#33279=ORIENTED_EDGE('',*,*,#23149,.T.);
#33280=ORIENTED_EDGE('',*,*,#23150,.T.);
#33281=ORIENTED_EDGE('',*,*,#23152,.T.);
#33282=ORIENTED_EDGE('',*,*,#23153,.F.);
#33283=ORIENTED_EDGE('',*,*,#23154,.F.);
#33284=ORIENTED_EDGE('',*,*,#23155,.F.);
#33285=ORIENTED_EDGE('',*,*,#23156,.T.);
#33286=ORIENTED_EDGE('',*,*,#23153,.T.);
#33287=ORIENTED_EDGE('',*,*,#23154,.T.);
#33288=ORIENTED_EDGE('',*,*,#23156,.F.);
#33289=ORIENTED_EDGE('',*,*,#23157,.F.);
#33290=ORIENTED_EDGE('',*,*,#23158,.T.);
#33291=ORIENTED_EDGE('',*,*,#23155,.T.);
#33292=ORIENTED_EDGE('',*,*,#23158,.F.);
#33293=ORIENTED_EDGE('',*,*,#23157,.T.);
#33294=ORIENTED_EDGE('',*,*,#23159,.F.);
#33295=ORIENTED_EDGE('',*,*,#23159,.T.);
#33296=ORIENTED_EDGE('',*,*,#23160,.T.);
#33297=ORIENTED_EDGE('',*,*,#23161,.F.);
#33298=ORIENTED_EDGE('',*,*,#23160,.F.);
#33299=ORIENTED_EDGE('',*,*,#23162,.F.);
#33300=ORIENTED_EDGE('',*,*,#23161,.T.);
#33301=ORIENTED_EDGE('',*,*,#23163,.F.);
#33302=ORIENTED_EDGE('',*,*,#23162,.T.);
#33303=ORIENTED_EDGE('',*,*,#23163,.T.);
#33304=ORIENTED_EDGE('',*,*,#23164,.F.);
#33305=ORIENTED_EDGE('',*,*,#23165,.F.);
#33306=ORIENTED_EDGE('',*,*,#23165,.T.);
#33307=ORIENTED_EDGE('',*,*,#23166,.T.);
#33308=ORIENTED_EDGE('',*,*,#23145,.F.);
#33309=ORIENTED_EDGE('',*,*,#23166,.F.);
#33310=ORIENTED_EDGE('',*,*,#23164,.T.);
#37770=CYLINDRICAL_SURFACE('',#43796,40.);
#37771=CYLINDRICAL_SURFACE('',#43801,41.);
#37772=CYLINDRICAL_SURFACE('',#43808,14.);
#37773=CYLINDRICAL_SURFACE('',#43812,12.);
#39609=ADVANCED_FACE('',(#3806),#37770,.F.);
#39610=ADVANCED_FACE('',(#3807,#1066),#1436,.T.);
#39611=ADVANCED_FACE('',(#3808),#37771,.T.);
#39612=ADVANCED_FACE('',(#3809),#1934,.T.);
#39613=ADVANCED_FACE('',(#3810),#687,.T.);
#39614=ADVANCED_FACE('',(#3811),#37772,.T.);
#39615=ADVANCED_FACE('',(#3812,#1067),#1437,.T.);
#39616=ADVANCED_FACE('',(#3813),#37773,.F.);
#39617=ADVANCED_FACE('',(#3814,#1068),#1438,.T.);
#39618=ADVANCED_FACE('',(#3815),#1935,.T.);
#39619=ADVANCED_FACE('',(#3816),#688,.F.);
#40351=CLOSED_SHELL('',(#39609,#39610,#39611,#39612,#39613,#39614,#39615,
#39616,#39617,#39618,#39619));
#43795=AXIS2_PLACEMENT_3D('',#81231,#53269,#53270);
#43796=AXIS2_PLACEMENT_3D('',#81232,#53271,#53272);
#43797=AXIS2_PLACEMENT_3D('',#81234,#53273,#53274);
#43798=AXIS2_PLACEMENT_3D('',#81237,#53276,#53277);
#43799=AXIS2_PLACEMENT_3D('',#81238,#53278,#53279);
#43800=AXIS2_PLACEMENT_3D('',#81240,#53280,#53281);
#43801=AXIS2_PLACEMENT_3D('',#81241,#53282,#53283);
#43802=AXIS2_PLACEMENT_3D('',#81244,#53284,#53285);
#43803=AXIS2_PLACEMENT_3D('',#81245,#53286,#53287);
#43804=AXIS2_PLACEMENT_3D('',#82099,#53289,#53290);
#43805=AXIS2_PLACEMENT_3D('',#82100,#53291,#53292);
#43806=AXIS2_PLACEMENT_3D('',#82101,#53293,#53294);
#43807=AXIS2_PLACEMENT_3D('',#82103,#53295,#53296);
#43808=AXIS2_PLACEMENT_3D('',#82105,#53298,#53299);
#43809=AXIS2_PLACEMENT_3D('',#82107,#53300,#53301);
#43810=AXIS2_PLACEMENT_3D('',#82109,#53303,#53304);
#43811=AXIS2_PLACEMENT_3D('',#82111,#53305,#53306);
#43812=AXIS2_PLACEMENT_3D('',#82112,#53307,#53308);
#43813=AXIS2_PLACEMENT_3D('',#82115,#53310,#53311);
#43814=AXIS2_PLACEMENT_3D('',#82116,#53312,#53313);
#43815=AXIS2_PLACEMENT_3D('',#82118,#53314,#53315);
#43816=AXIS2_PLACEMENT_3D('',#82971,#53316,#53317);
#43817=AXIS2_PLACEMENT_3D('',#82972,#53318,#53319);
#43818=AXIS2_PLACEMENT_3D('',#82973,#53320,#53321);
#53269=DIRECTION('axis',(0.,0.,1.));
#53270=DIRECTION('refdir',(1.,0.,0.));
#53271=DIRECTION('center_axis',(1.,0.,0.));
#53272=DIRECTION('ref_axis',(0.,1.,0.));
#53273=DIRECTION('center_axis',(1.,0.,0.));
#53274=DIRECTION('ref_axis',(0.,0.,-1.));
#53275=DIRECTION('',(-1.,0.,0.));
#53276=DIRECTION('center_axis',(1.,0.,0.));
#53277=DIRECTION('ref_axis',(0.,0.,-1.));
#53278=DIRECTION('center_axis',(-1.,0.,0.));
#53279=DIRECTION('ref_axis',(0.,0.,1.));
#53280=DIRECTION('center_axis',(1.,0.,0.));
#53281=DIRECTION('ref_axis',(0.,0.,-1.));
#53282=DIRECTION('center_axis',(1.,0.,0.));
#53283=DIRECTION('ref_axis',(0.,1.,0.));
#53284=DIRECTION('center_axis',(1.,0.,0.));
#53285=DIRECTION('ref_axis',(0.,0.,-1.));
#53286=DIRECTION('center_axis',(1.,0.,0.));
#53287=DIRECTION('ref_axis',(0.,0.,-1.));
#53288=DIRECTION('',(-1.,0.,0.));
#53289=DIRECTION('center_axis',(1.,0.,0.));
#53290=DIRECTION('ref_axis',(0.,0.,-1.));
#53291=DIRECTION('center_axis',(1.,0.,0.));
#53292=DIRECTION('ref_axis',(0.,0.,-1.));
#53293=DIRECTION('center_axis',(-1.,0.,0.));
#53294=DIRECTION('ref_axis',(0.,1.,0.));
#53295=DIRECTION('center_axis',(1.,0.,0.));
#53296=DIRECTION('ref_axis',(0.,0.,-1.));
#53297=DIRECTION('',(-0.371390676354097,-0.928476690885262,-1.13705600757556E-16));
#53298=DIRECTION('center_axis',(1.,0.,0.));
#53299=DIRECTION('ref_axis',(0.,1.,0.));
#53300=DIRECTION('center_axis',(1.,0.,0.));
#53301=DIRECTION('ref_axis',(0.,0.,-1.));
#53302=DIRECTION('',(-1.,0.,0.));
#53303=DIRECTION('center_axis',(1.,0.,0.));
#53304=DIRECTION('ref_axis',(0.,0.,-1.));
#53305=DIRECTION('center_axis',(1.,0.,0.));
#53306=DIRECTION('ref_axis',(0.,0.,-1.));
#53307=DIRECTION('center_axis',(1.,0.,0.));
#53308=DIRECTION('ref_axis',(0.,1.,0.));
#53309=DIRECTION('',(-1.,0.,0.));
#53310=DIRECTION('center_axis',(1.,0.,0.));
#53311=DIRECTION('ref_axis',(0.,0.,-1.));
#53312=DIRECTION('center_axis',(-1.,0.,0.));
#53313=DIRECTION('ref_axis',(0.,0.,1.));
#53314=DIRECTION('center_axis',(1.,0.,0.));
#53315=DIRECTION('ref_axis',(0.,0.,-1.));
#53316=DIRECTION('center_axis',(1.,0.,0.));
#53317=DIRECTION('ref_axis',(0.,0.,-1.));
#53318=DIRECTION('center_axis',(1.,0.,0.));
#53319=DIRECTION('ref_axis',(0.,0.,-1.));
#53320=DIRECTION('center_axis',(-1.,0.,0.));
#53321=DIRECTION('ref_axis',(0.,1.,0.));
#53322=DIRECTION('',(-0.316227766016822,-0.948683298050519,-1.16180196436212E-16));
#81231=CARTESIAN_POINT('',(0.,0.,0.));
#81232=CARTESIAN_POINT('Origin',(159.,0.,0.));
#81233=CARTESIAN_POINT('',(166.,-40.,-4.89858719658941E-15));
#81234=CARTESIAN_POINT('Origin',(166.,0.,0.));
#81235=CARTESIAN_POINT('',(152.,-40.,-4.89858719658941E-15));
#81236=CARTESIAN_POINT('',(159.,-40.,-4.89858719658941E-15));
#81237=CARTESIAN_POINT('Origin',(152.,0.,0.));
#81238=CARTESIAN_POINT('Origin',(152.,41.,0.));
#81239=CARTESIAN_POINT('',(152.,-41.,-5.02105187650415E-15));
#81240=CARTESIAN_POINT('Origin',(152.,0.,0.));
#81241=CARTESIAN_POINT('Origin',(159.,0.,0.));
#81242=CARTESIAN_POINT('',(166.,41.,0.));
#81243=CARTESIAN_POINT('',(166.,-41.,-5.02105187650415E-15));
#81244=CARTESIAN_POINT('Origin',(166.,0.,0.));
#81245=CARTESIAN_POINT('Origin',(166.,0.,0.));
#81246=CARTESIAN_POINT('',(159.,-41.,-5.02105187650415E-15));
#81247=CARTESIAN_POINT('Ctrl Pts',(216.,16.5,0.));
#81248=CARTESIAN_POINT('Ctrl Pts',(216.,16.5,16.5));
#81249=CARTESIAN_POINT('Ctrl Pts',(216.,0.,16.5));
#81250=CARTESIAN_POINT('Ctrl Pts',(216.,-16.5,16.5));
#81251=CARTESIAN_POINT('Ctrl Pts',(216.,-16.5,0.));
#81252=CARTESIAN_POINT('Ctrl Pts',(216.,-16.5,-16.5));
#81253=CARTESIAN_POINT('Ctrl Pts',(216.,0.,-16.5));
#81254=CARTESIAN_POINT('Ctrl Pts',(216.,16.5,-16.5));
#81255=CARTESIAN_POINT('Ctrl Pts',(216.,16.5,0.));
#81256=CARTESIAN_POINT('Ctrl Pts',(215.931357948425,16.5650312142703,0.));
#81257=CARTESIAN_POINT('Ctrl Pts',(215.931357948425,16.5650312142703,16.5650312142703));
#81258=CARTESIAN_POINT('Ctrl Pts',(215.931357948425,0.,16.5650312142703));
#81259=CARTESIAN_POINT('Ctrl Pts',(215.931357948425,-16.5650312142703,16.5650312142703));
#81260=CARTESIAN_POINT('Ctrl Pts',(215.931357948425,-16.5650312142703,0.));
#81261=CARTESIAN_POINT('Ctrl Pts',(215.931357948425,-16.5650312142703,-16.5650312142703));
#81262=CARTESIAN_POINT('Ctrl Pts',(215.931357948425,0.,-16.5650312142703));
#81263=CARTESIAN_POINT('Ctrl Pts',(215.931357948425,16.5650312142703,-16.5650312142703));
#81264=CARTESIAN_POINT('Ctrl Pts',(215.931357948425,16.5650312142703,0.));
#81265=CARTESIAN_POINT('Ctrl Pts',(215.790485987678,16.7090430293136,0.));
#81266=CARTESIAN_POINT('Ctrl Pts',(215.790485987678,16.7090430293136,16.7090430293136));
#81267=CARTESIAN_POINT('Ctrl Pts',(215.790485987678,0.,16.7090430293136));
#81268=CARTESIAN_POINT('Ctrl Pts',(215.790485987678,-16.7090430293136,16.7090430293136));
#81269=CARTESIAN_POINT('Ctrl Pts',(215.790485987678,-16.7090430293136,0.));
#81270=CARTESIAN_POINT('Ctrl Pts',(215.790485987678,-16.7090430293136,-16.7090430293136));
#81271=CARTESIAN_POINT('Ctrl Pts',(215.790485987678,0.,-16.7090430293136));
#81272=CARTESIAN_POINT('Ctrl Pts',(215.790485987678,16.7090430293136,-16.7090430293136));
#81273=CARTESIAN_POINT('Ctrl Pts',(215.790485987678,16.7090430293136,0.));
#81274=CARTESIAN_POINT('Ctrl Pts',(215.568414172701,16.9669101302242,0.));
#81275=CARTESIAN_POINT('Ctrl Pts',(215.568414172701,16.9669101302242,16.9669101302242));
#81276=CARTESIAN_POINT('Ctrl Pts',(215.568414172701,0.,16.9669101302242));
#81277=CARTESIAN_POINT('Ctrl Pts',(215.568414172701,-16.9669101302242,16.9669101302242));
#81278=CARTESIAN_POINT('Ctrl Pts',(215.568414172701,-16.9669101302242,0.));
#81279=CARTESIAN_POINT('Ctrl Pts',(215.568414172701,-16.9669101302242,-16.9669101302242));
#81280=CARTESIAN_POINT('Ctrl Pts',(215.568414172701,0.,-16.9669101302242));
#81281=CARTESIAN_POINT('Ctrl Pts',(215.568414172701,16.9669101302242,-16.9669101302242));
#81282=CARTESIAN_POINT('Ctrl Pts',(215.568414172701,16.9669101302242,0.));
#81283=CARTESIAN_POINT('Ctrl Pts',(215.250787804816,17.3944424189593,0.));
#81284=CARTESIAN_POINT('Ctrl Pts',(215.250787804816,17.3944424189593,17.3944424189593));
#81285=CARTESIAN_POINT('Ctrl Pts',(215.250787804816,0.,17.3944424189593));
#81286=CARTESIAN_POINT('Ctrl Pts',(215.250787804816,-17.3944424189593,17.3944424189593));
#81287=CARTESIAN_POINT('Ctrl Pts',(215.250787804816,-17.3944424189593,0.));
#81288=CARTESIAN_POINT('Ctrl Pts',(215.250787804816,-17.3944424189593,-17.3944424189593));
#81289=CARTESIAN_POINT('Ctrl Pts',(215.250787804816,0.,-17.3944424189593));
#81290=CARTESIAN_POINT('Ctrl Pts',(215.250787804816,17.3944424189593,-17.3944424189593));
#81291=CARTESIAN_POINT('Ctrl Pts',(215.250787804816,17.3944424189593,0.));
#81292=CARTESIAN_POINT('Ctrl Pts',(214.818499221249,18.0645628079122,0.));
#81293=CARTESIAN_POINT('Ctrl Pts',(214.818499221249,18.0645628079122,18.0645628079122));
#81294=CARTESIAN_POINT('Ctrl Pts',(214.818499221249,0.,18.0645628079122));
#81295=CARTESIAN_POINT('Ctrl Pts',(214.818499221249,-18.0645628079122,18.0645628079122));
#81296=CARTESIAN_POINT('Ctrl Pts',(214.818499221249,-18.0645628079122,0.));
#81297=CARTESIAN_POINT('Ctrl Pts',(214.818499221249,-18.0645628079122,-18.0645628079122));
#81298=CARTESIAN_POINT('Ctrl Pts',(214.818499221249,0.,-18.0645628079122));
#81299=CARTESIAN_POINT('Ctrl Pts',(214.818499221249,18.0645628079122,-18.0645628079122));
#81300=CARTESIAN_POINT('Ctrl Pts',(214.818499221249,18.0645628079122,0.));
#81301=CARTESIAN_POINT('Ctrl Pts',(214.352945230993,18.8585426236962,0.));
#81302=CARTESIAN_POINT('Ctrl Pts',(214.352945230993,18.8585426236962,18.8585426236962));
#81303=CARTESIAN_POINT('Ctrl Pts',(214.352945230993,0.,18.8585426236962));
#81304=CARTESIAN_POINT('Ctrl Pts',(214.352945230993,-18.8585426236962,18.8585426236962));
#81305=CARTESIAN_POINT('Ctrl Pts',(214.352945230993,-18.8585426236962,0.));
#81306=CARTESIAN_POINT('Ctrl Pts',(214.352945230993,-18.8585426236962,-18.8585426236962));
#81307=CARTESIAN_POINT('Ctrl Pts',(214.352945230993,0.,-18.8585426236962));
#81308=CARTESIAN_POINT('Ctrl Pts',(214.352945230993,18.8585426236962,-18.8585426236962));
#81309=CARTESIAN_POINT('Ctrl Pts',(214.352945230993,18.8585426236962,0.));
#81310=CARTESIAN_POINT('Ctrl Pts',(213.858063274574,19.7528683772512,0.));
#81311=CARTESIAN_POINT('Ctrl Pts',(213.858063274574,19.7528683772512,19.7528683772512));
#81312=CARTESIAN_POINT('Ctrl Pts',(213.858063274574,0.,19.7528683772512));
#81313=CARTESIAN_POINT('Ctrl Pts',(213.858063274574,-19.7528683772512,19.7528683772512));
#81314=CARTESIAN_POINT('Ctrl Pts',(213.858063274574,-19.7528683772512,0.));
#81315=CARTESIAN_POINT('Ctrl Pts',(213.858063274574,-19.7528683772512,-19.7528683772512));
#81316=CARTESIAN_POINT('Ctrl Pts',(213.858063274574,0.,-19.7528683772512));
#81317=CARTESIAN_POINT('Ctrl Pts',(213.858063274574,19.7528683772512,-19.7528683772512));
#81318=CARTESIAN_POINT('Ctrl Pts',(213.858063274574,19.7528683772512,0.));
#81319=CARTESIAN_POINT('Ctrl Pts',(213.340647821643,20.70741247154,0.));
#81320=CARTESIAN_POINT('Ctrl Pts',(213.340647821643,20.70741247154,20.70741247154));
#81321=CARTESIAN_POINT('Ctrl Pts',(213.340647821643,0.,20.70741247154));
#81322=CARTESIAN_POINT('Ctrl Pts',(213.340647821643,-20.70741247154,20.70741247154));
#81323=CARTESIAN_POINT('Ctrl Pts',(213.340647821643,-20.70741247154,0.));
#81324=CARTESIAN_POINT('Ctrl Pts',(213.340647821643,-20.70741247154,-20.70741247154));
#81325=CARTESIAN_POINT('Ctrl Pts',(213.340647821643,0.,-20.70741247154));
#81326=CARTESIAN_POINT('Ctrl Pts',(213.340647821643,20.70741247154,-20.70741247154));
#81327=CARTESIAN_POINT('Ctrl Pts',(213.340647821643,20.70741247154,0.));
#81328=CARTESIAN_POINT('Ctrl Pts',(212.810267068812,21.6644655526099,0.));
#81329=CARTESIAN_POINT('Ctrl Pts',(212.810267068812,21.6644655526099,21.6644655526099));
#81330=CARTESIAN_POINT('Ctrl Pts',(212.810267068812,0.,21.6644655526099));
#81331=CARTESIAN_POINT('Ctrl Pts',(212.810267068812,-21.6644655526099,21.6644655526099));
#81332=CARTESIAN_POINT('Ctrl Pts',(212.810267068812,-21.6644655526099,0.));
#81333=CARTESIAN_POINT('Ctrl Pts',(212.810267068812,-21.6644655526099,-21.6644655526099));
#81334=CARTESIAN_POINT('Ctrl Pts',(212.810267068812,0.,-21.6644655526099));
#81335=CARTESIAN_POINT('Ctrl Pts',(212.810267068812,21.6644655526099,-21.6644655526099));
#81336=CARTESIAN_POINT('Ctrl Pts',(212.810267068812,21.6644655526099,0.));
#81337=CARTESIAN_POINT('Ctrl Pts',(212.2765623513,22.557779972217,0.));
#81338=CARTESIAN_POINT('Ctrl Pts',(212.2765623513,22.5577799722169,22.5577799722169));
#81339=CARTESIAN_POINT('Ctrl Pts',(212.2765623513,0.,22.557779972217));
#81340=CARTESIAN_POINT('Ctrl Pts',(212.2765623513,-22.5577799722169,22.5577799722169));
#81341=CARTESIAN_POINT('Ctrl Pts',(212.2765623513,-22.557779972217,0.));
#81342=CARTESIAN_POINT('Ctrl Pts',(212.2765623513,-22.5577799722169,-22.5577799722169));
#81343=CARTESIAN_POINT('Ctrl Pts',(212.2765623513,0.,-22.557779972217));
#81344=CARTESIAN_POINT('Ctrl Pts',(212.2765623513,22.5577799722169,-22.5577799722169));
#81345=CARTESIAN_POINT('Ctrl Pts',(212.2765623513,22.557779972217,0.));
#81346=CARTESIAN_POINT('Ctrl Pts',(211.747183985356,23.3196384840519,0.));
#81347=CARTESIAN_POINT('Ctrl Pts',(211.747183985356,23.3196384840519,23.3196384840519));
#81348=CARTESIAN_POINT('Ctrl Pts',(211.747183985356,0.,23.3196384840519));
#81349=CARTESIAN_POINT('Ctrl Pts',(211.747183985356,-23.3196384840519,23.3196384840519));
#81350=CARTESIAN_POINT('Ctrl Pts',(211.747183985356,-23.3196384840519,0.));
#81351=CARTESIAN_POINT('Ctrl Pts',(211.747183985356,-23.3196384840519,-23.3196384840519));
#81352=CARTESIAN_POINT('Ctrl Pts',(211.747183985356,0.,-23.3196384840519));
#81353=CARTESIAN_POINT('Ctrl Pts',(211.747183985356,23.3196384840519,-23.3196384840519));
#81354=CARTESIAN_POINT('Ctrl Pts',(211.747183985356,23.3196384840519,0.));
#81355=CARTESIAN_POINT('Ctrl Pts',(211.225193342687,23.8887926005784,0.));
#81356=CARTESIAN_POINT('Ctrl Pts',(211.225193342687,23.8887926005784,23.8887926005784));
#81357=CARTESIAN_POINT('Ctrl Pts',(211.225193342687,0.,23.8887926005784));
#81358=CARTESIAN_POINT('Ctrl Pts',(211.225193342687,-23.8887926005784,23.8887926005784));
#81359=CARTESIAN_POINT('Ctrl Pts',(211.225193342687,-23.8887926005784,0.));
#81360=CARTESIAN_POINT('Ctrl Pts',(211.225193342687,-23.8887926005784,-23.8887926005784));
#81361=CARTESIAN_POINT('Ctrl Pts',(211.225193342687,0.,-23.8887926005784));
#81362=CARTESIAN_POINT('Ctrl Pts',(211.225193342687,23.8887926005784,-23.8887926005784));
#81363=CARTESIAN_POINT('Ctrl Pts',(211.225193342687,23.8887926005784,0.));
#81364=CARTESIAN_POINT('Ctrl Pts',(210.707332937096,24.2178287727218,0.));
#81365=CARTESIAN_POINT('Ctrl Pts',(210.707332937096,24.2178287727218,24.2178287727218));
#81366=CARTESIAN_POINT('Ctrl Pts',(210.707332937096,0.,24.2178287727218));
#81367=CARTESIAN_POINT('Ctrl Pts',(210.707332937096,-24.2178287727218,24.2178287727218));
#81368=CARTESIAN_POINT('Ctrl Pts',(210.707332937096,-24.2178287727218,0.));
#81369=CARTESIAN_POINT('Ctrl Pts',(210.707332937096,-24.2178287727218,-24.2178287727218));
#81370=CARTESIAN_POINT('Ctrl Pts',(210.707332937096,0.,-24.2178287727218));
#81371=CARTESIAN_POINT('Ctrl Pts',(210.707332937096,24.2178287727218,-24.2178287727218));
#81372=CARTESIAN_POINT('Ctrl Pts',(210.707332937096,24.2178287727218,0.));
#81373=CARTESIAN_POINT('Ctrl Pts',(210.180310680863,24.2813063241724,0.));
#81374=CARTESIAN_POINT('Ctrl Pts',(210.180310680863,24.2813063241724,24.2813063241724));
#81375=CARTESIAN_POINT('Ctrl Pts',(210.180310680863,0.,24.2813063241724));
#81376=CARTESIAN_POINT('Ctrl Pts',(210.180310680863,-24.2813063241724,24.2813063241724));
#81377=CARTESIAN_POINT('Ctrl Pts',(210.180310680863,-24.2813063241724,0.));
#81378=CARTESIAN_POINT('Ctrl Pts',(210.180310680863,-24.2813063241724,-24.2813063241724));
#81379=CARTESIAN_POINT('Ctrl Pts',(210.180310680863,0.,-24.2813063241724));
#81380=CARTESIAN_POINT('Ctrl Pts',(210.180310680863,24.2813063241724,-24.2813063241724));
#81381=CARTESIAN_POINT('Ctrl Pts',(210.180310680863,24.2813063241724,0.));
#81382=CARTESIAN_POINT('Ctrl Pts',(209.624909485776,24.0813843942427,0.));
#81383=CARTESIAN_POINT('Ctrl Pts',(209.624909485776,24.0813843942427,24.0813843942427));
#81384=CARTESIAN_POINT('Ctrl Pts',(209.624909485776,0.,24.0813843942427));
#81385=CARTESIAN_POINT('Ctrl Pts',(209.624909485776,-24.0813843942427,24.0813843942427));
#81386=CARTESIAN_POINT('Ctrl Pts',(209.624909485776,-24.0813843942427,0.));
#81387=CARTESIAN_POINT('Ctrl Pts',(209.624909485776,-24.0813843942427,-24.0813843942427));
#81388=CARTESIAN_POINT('Ctrl Pts',(209.624909485776,0.,-24.0813843942427));
#81389=CARTESIAN_POINT('Ctrl Pts',(209.624909485776,24.0813843942427,-24.0813843942427));
#81390=CARTESIAN_POINT('Ctrl Pts',(209.624909485776,24.0813843942427,0.));
#81391=CARTESIAN_POINT('Ctrl Pts',(209.02608343001,23.651711850736,0.));
#81392=CARTESIAN_POINT('Ctrl Pts',(209.02608343001,23.651711850736,23.651711850736));
#81393=CARTESIAN_POINT('Ctrl Pts',(209.02608343001,0.,23.651711850736));
#81394=CARTESIAN_POINT('Ctrl Pts',(209.02608343001,-23.651711850736,23.651711850736));
#81395=CARTESIAN_POINT('Ctrl Pts',(209.02608343001,-23.651711850736,0.));
#81396=CARTESIAN_POINT('Ctrl Pts',(209.02608343001,-23.651711850736,-23.651711850736));
#81397=CARTESIAN_POINT('Ctrl Pts',(209.02608343001,0.,-23.651711850736));
#81398=CARTESIAN_POINT('Ctrl Pts',(209.02608343001,23.651711850736,-23.651711850736));
#81399=CARTESIAN_POINT('Ctrl Pts',(209.02608343001,23.651711850736,0.));
#81400=CARTESIAN_POINT('Ctrl Pts',(208.381214512496,23.0617114361388,0.));
#81401=CARTESIAN_POINT('Ctrl Pts',(208.381214512496,23.0617114361388,23.0617114361388));
#81402=CARTESIAN_POINT('Ctrl Pts',(208.381214512496,0.,23.0617114361388));
#81403=CARTESIAN_POINT('Ctrl Pts',(208.381214512496,-23.0617114361388,23.0617114361388));
#81404=CARTESIAN_POINT('Ctrl Pts',(208.381214512496,-23.0617114361388,0.));
#81405=CARTESIAN_POINT('Ctrl Pts',(208.381214512496,-23.0617114361388,-23.0617114361388));
#81406=CARTESIAN_POINT('Ctrl Pts',(208.381214512496,0.,-23.0617114361388));
#81407=CARTESIAN_POINT('Ctrl Pts',(208.381214512496,23.0617114361388,-23.0617114361388));
#81408=CARTESIAN_POINT('Ctrl Pts',(208.381214512496,23.0617114361388,0.));
#81409=CARTESIAN_POINT('Ctrl Pts',(207.709418184682,22.4211128317459,0.));
#81410=CARTESIAN_POINT('Ctrl Pts',(207.709418184682,22.4211128317459,22.4211128317459));
#81411=CARTESIAN_POINT('Ctrl Pts',(207.709418184682,0.,22.4211128317459));
#81412=CARTESIAN_POINT('Ctrl Pts',(207.709418184682,-22.4211128317459,22.4211128317459));
#81413=CARTESIAN_POINT('Ctrl Pts',(207.709418184682,-22.4211128317459,0.));
#81414=CARTESIAN_POINT('Ctrl Pts',(207.709418184682,-22.4211128317459,-22.4211128317459));
#81415=CARTESIAN_POINT('Ctrl Pts',(207.709418184682,0.,-22.4211128317459));
#81416=CARTESIAN_POINT('Ctrl Pts',(207.709418184682,22.4211128317459,-22.4211128317459));
#81417=CARTESIAN_POINT('Ctrl Pts',(207.709418184682,22.4211128317459,0.));
#81418=CARTESIAN_POINT('Ctrl Pts',(207.042444432711,21.858011778557,0.));
#81419=CARTESIAN_POINT('Ctrl Pts',(207.042444432711,21.858011778557,21.858011778557));
#81420=CARTESIAN_POINT('Ctrl Pts',(207.042444432711,0.,21.858011778557));
#81421=CARTESIAN_POINT('Ctrl Pts',(207.042444432711,-21.858011778557,21.858011778557));
#81422=CARTESIAN_POINT('Ctrl Pts',(207.042444432711,-21.858011778557,0.));
#81423=CARTESIAN_POINT('Ctrl Pts',(207.042444432711,-21.858011778557,-21.858011778557));
#81424=CARTESIAN_POINT('Ctrl Pts',(207.042444432711,0.,-21.858011778557));
#81425=CARTESIAN_POINT('Ctrl Pts',(207.042444432711,21.858011778557,-21.858011778557));
#81426=CARTESIAN_POINT('Ctrl Pts',(207.042444432711,21.858011778557,0.));
#81427=CARTESIAN_POINT('Ctrl Pts',(206.415057633172,21.495656810279,0.));
#81428=CARTESIAN_POINT('Ctrl Pts',(206.415057633172,21.495656810279,21.495656810279));
#81429=CARTESIAN_POINT('Ctrl Pts',(206.415057633172,0.,21.495656810279));
#81430=CARTESIAN_POINT('Ctrl Pts',(206.415057633172,-21.495656810279,21.495656810279));
#81431=CARTESIAN_POINT('Ctrl Pts',(206.415057633172,-21.495656810279,0.));
#81432=CARTESIAN_POINT('Ctrl Pts',(206.415057633172,-21.495656810279,-21.495656810279));
#81433=CARTESIAN_POINT('Ctrl Pts',(206.415057633172,0.,-21.495656810279));
#81434=CARTESIAN_POINT('Ctrl Pts',(206.415057633172,21.495656810279,-21.495656810279));
#81435=CARTESIAN_POINT('Ctrl Pts',(206.415057633172,21.495656810279,0.));
#81436=CARTESIAN_POINT('Ctrl Pts',(205.856117010386,21.4309931834381,0.));
#81437=CARTESIAN_POINT('Ctrl Pts',(205.856117010386,21.4309931834381,21.4309931834381));
#81438=CARTESIAN_POINT('Ctrl Pts',(205.856117010386,0.,21.4309931834381));
#81439=CARTESIAN_POINT('Ctrl Pts',(205.856117010386,-21.4309931834381,21.4309931834381));
#81440=CARTESIAN_POINT('Ctrl Pts',(205.856117010386,-21.4309931834381,0.));
#81441=CARTESIAN_POINT('Ctrl Pts',(205.856117010386,-21.4309931834381,-21.4309931834381));
#81442=CARTESIAN_POINT('Ctrl Pts',(205.856117010386,0.,-21.4309931834381));
#81443=CARTESIAN_POINT('Ctrl Pts',(205.856117010386,21.4309931834381,-21.4309931834381));
#81444=CARTESIAN_POINT('Ctrl Pts',(205.856117010386,21.4309931834381,0.));
#81445=CARTESIAN_POINT('Ctrl Pts',(205.378164090918,21.7094404040115,0.));
#81446=CARTESIAN_POINT('Ctrl Pts',(205.378164090918,21.7094404040115,21.7094404040115));
#81447=CARTESIAN_POINT('Ctrl Pts',(205.378164090918,0.,21.7094404040115));
#81448=CARTESIAN_POINT('Ctrl Pts',(205.378164090918,-21.7094404040115,21.7094404040115));
#81449=CARTESIAN_POINT('Ctrl Pts',(205.378164090918,-21.7094404040115,0.));
#81450=CARTESIAN_POINT('Ctrl Pts',(205.378164090918,-21.7094404040115,-21.7094404040115));
#81451=CARTESIAN_POINT('Ctrl Pts',(205.378164090918,0.,-21.7094404040115));
#81452=CARTESIAN_POINT('Ctrl Pts',(205.378164090918,21.7094404040115,-21.7094404040115));
#81453=CARTESIAN_POINT('Ctrl Pts',(205.378164090918,21.7094404040115,0.));
#81454=CARTESIAN_POINT('Ctrl Pts',(204.97132698008,22.3105170035492,0.));
#81455=CARTESIAN_POINT('Ctrl Pts',(204.97132698008,22.3105170035492,22.3105170035492));
#81456=CARTESIAN_POINT('Ctrl Pts',(204.97132698008,0.,22.3105170035492));
#81457=CARTESIAN_POINT('Ctrl Pts',(204.97132698008,-22.3105170035492,22.3105170035492));
#81458=CARTESIAN_POINT('Ctrl Pts',(204.97132698008,-22.3105170035492,0.));
#81459=CARTESIAN_POINT('Ctrl Pts',(204.97132698008,-22.3105170035492,-22.3105170035492));
#81460=CARTESIAN_POINT('Ctrl Pts',(204.97132698008,0.,-22.3105170035492));
#81461=CARTESIAN_POINT('Ctrl Pts',(204.97132698008,22.3105170035492,-22.3105170035492));
#81462=CARTESIAN_POINT('Ctrl Pts',(204.97132698008,22.3105170035492,0.));
#81463=CARTESIAN_POINT('Ctrl Pts',(204.611869907935,23.1702821776947,0.));
#81464=CARTESIAN_POINT('Ctrl Pts',(204.611869907935,23.1702821776947,23.1702821776947));
#81465=CARTESIAN_POINT('Ctrl Pts',(204.611869907935,0.,23.1702821776947));
#81466=CARTESIAN_POINT('Ctrl Pts',(204.611869907935,-23.1702821776947,23.1702821776947));
#81467=CARTESIAN_POINT('Ctrl Pts',(204.611869907935,-23.1702821776947,0.));
#81468=CARTESIAN_POINT('Ctrl Pts',(204.611869907935,-23.1702821776947,-23.1702821776947));
#81469=CARTESIAN_POINT('Ctrl Pts',(204.611869907935,0.,-23.1702821776947));
#81470=CARTESIAN_POINT('Ctrl Pts',(204.611869907935,23.1702821776947,-23.1702821776947));
#81471=CARTESIAN_POINT('Ctrl Pts',(204.611869907935,23.1702821776947,0.));
#81472=CARTESIAN_POINT('Ctrl Pts',(204.268492247486,24.1981104944312,0.));
#81473=CARTESIAN_POINT('Ctrl Pts',(204.268492247486,24.1981104944312,24.1981104944312));
#81474=CARTESIAN_POINT('Ctrl Pts',(204.268492247486,0.,24.1981104944312));
#81475=CARTESIAN_POINT('Ctrl Pts',(204.268492247486,-24.1981104944312,24.1981104944312));
#81476=CARTESIAN_POINT('Ctrl Pts',(204.268492247486,-24.1981104944312,0.));
#81477=CARTESIAN_POINT('Ctrl Pts',(204.268492247486,-24.1981104944312,-24.1981104944312));
#81478=CARTESIAN_POINT('Ctrl Pts',(204.268492247486,0.,-24.1981104944312));
#81479=CARTESIAN_POINT('Ctrl Pts',(204.268492247486,24.1981104944312,-24.1981104944312));
#81480=CARTESIAN_POINT('Ctrl Pts',(204.268492247486,24.1981104944312,0.));
#81481=CARTESIAN_POINT('Ctrl Pts',(203.909197365198,25.2948962814451,0.));
#81482=CARTESIAN_POINT('Ctrl Pts',(203.909197365198,25.2948962814451,25.2948962814451));
#81483=CARTESIAN_POINT('Ctrl Pts',(203.909197365198,0.,25.2948962814451));
#81484=CARTESIAN_POINT('Ctrl Pts',(203.909197365198,-25.2948962814451,25.2948962814451));
#81485=CARTESIAN_POINT('Ctrl Pts',(203.909197365198,-25.2948962814451,0.));
#81486=CARTESIAN_POINT('Ctrl Pts',(203.909197365198,-25.2948962814451,-25.2948962814451));
#81487=CARTESIAN_POINT('Ctrl Pts',(203.909197365198,0.,-25.2948962814451));
#81488=CARTESIAN_POINT('Ctrl Pts',(203.909197365198,25.2948962814451,-25.2948962814451));
#81489=CARTESIAN_POINT('Ctrl Pts',(203.909197365198,25.2948962814451,0.));
#81490=CARTESIAN_POINT('Ctrl Pts',(203.508634483801,26.3724343604023,0.));
#81491=CARTESIAN_POINT('Ctrl Pts',(203.508634483801,26.3724343604023,26.3724343604023));
#81492=CARTESIAN_POINT('Ctrl Pts',(203.508634483801,0.,26.3724343604023));
#81493=CARTESIAN_POINT('Ctrl Pts',(203.508634483801,-26.3724343604023,26.3724343604023));
#81494=CARTESIAN_POINT('Ctrl Pts',(203.508634483801,-26.3724343604023,0.));
#81495=CARTESIAN_POINT('Ctrl Pts',(203.508634483801,-26.3724343604023,-26.3724343604023));
#81496=CARTESIAN_POINT('Ctrl Pts',(203.508634483801,0.,-26.3724343604023));
#81497=CARTESIAN_POINT('Ctrl Pts',(203.508634483801,26.3724343604023,-26.3724343604023));
#81498=CARTESIAN_POINT('Ctrl Pts',(203.508634483801,26.3724343604023,0.));
#81499=CARTESIAN_POINT('Ctrl Pts',(203.052959516359,27.3665743841578,0.));
#81500=CARTESIAN_POINT('Ctrl Pts',(203.052959516359,27.3665743841578,27.3665743841578));
#81501=CARTESIAN_POINT('Ctrl Pts',(203.052959516359,0.,27.3665743841578));
#81502=CARTESIAN_POINT('Ctrl Pts',(203.052959516359,-27.3665743841578,27.3665743841578));
#81503=CARTESIAN_POINT('Ctrl Pts',(203.052959516359,-27.3665743841578,0.));
#81504=CARTESIAN_POINT('Ctrl Pts',(203.052959516359,-27.3665743841578,-27.3665743841578));
#81505=CARTESIAN_POINT('Ctrl Pts',(203.052959516359,0.,-27.3665743841578));
#81506=CARTESIAN_POINT('Ctrl Pts',(203.052959516359,27.3665743841578,-27.3665743841578));
#81507=CARTESIAN_POINT('Ctrl Pts',(203.052959516359,27.3665743841578,0.));
#81508=CARTESIAN_POINT('Ctrl Pts',(202.537022078747,28.231020604859,0.));
#81509=CARTESIAN_POINT('Ctrl Pts',(202.537022078747,28.231020604859,28.231020604859));
#81510=CARTESIAN_POINT('Ctrl Pts',(202.537022078747,0.,28.231020604859));
#81511=CARTESIAN_POINT('Ctrl Pts',(202.537022078747,-28.231020604859,28.231020604859));
#81512=CARTESIAN_POINT('Ctrl Pts',(202.537022078747,-28.231020604859,0.));
#81513=CARTESIAN_POINT('Ctrl Pts',(202.537022078747,-28.231020604859,-28.231020604859));
#81514=CARTESIAN_POINT('Ctrl Pts',(202.537022078747,0.,-28.231020604859));
#81515=CARTESIAN_POINT('Ctrl Pts',(202.537022078747,28.231020604859,-28.231020604859));
#81516=CARTESIAN_POINT('Ctrl Pts',(202.537022078747,28.231020604859,0.));
#81517=CARTESIAN_POINT('Ctrl Pts',(201.962968334053,28.934797520153,0.));
#81518=CARTESIAN_POINT('Ctrl Pts',(201.962968334053,28.934797520153,28.934797520153));
#81519=CARTESIAN_POINT('Ctrl Pts',(201.962968334053,0.,28.934797520153));
#81520=CARTESIAN_POINT('Ctrl Pts',(201.962968334053,-28.934797520153,28.934797520153));
#81521=CARTESIAN_POINT('Ctrl Pts',(201.962968334053,-28.934797520153,0.));
#81522=CARTESIAN_POINT('Ctrl Pts',(201.962968334053,-28.934797520153,-28.934797520153));
#81523=CARTESIAN_POINT('Ctrl Pts',(201.962968334053,0.,-28.934797520153));
#81524=CARTESIAN_POINT('Ctrl Pts',(201.962968334053,28.934797520153,-28.934797520153));
#81525=CARTESIAN_POINT('Ctrl Pts',(201.962968334053,28.934797520153,0.));
#81526=CARTESIAN_POINT('Ctrl Pts',(201.338274525702,29.4580312858847,0.));
#81527=CARTESIAN_POINT('Ctrl Pts',(201.338274525702,29.4580312858847,29.4580312858847));
#81528=CARTESIAN_POINT('Ctrl Pts',(201.338274525702,0.,29.4580312858847));
#81529=CARTESIAN_POINT('Ctrl Pts',(201.338274525702,-29.4580312858847,29.4580312858847));
#81530=CARTESIAN_POINT('Ctrl Pts',(201.338274525702,-29.4580312858847,0.));
#81531=CARTESIAN_POINT('Ctrl Pts',(201.338274525702,-29.4580312858847,-29.4580312858847));
#81532=CARTESIAN_POINT('Ctrl Pts',(201.338274525702,0.,-29.4580312858847));
#81533=CARTESIAN_POINT('Ctrl Pts',(201.338274525702,29.4580312858847,-29.4580312858847));
#81534=CARTESIAN_POINT('Ctrl Pts',(201.338274525702,29.4580312858847,0.));
#81535=CARTESIAN_POINT('Ctrl Pts',(200.674069577301,29.7890397540896,0.));
#81536=CARTESIAN_POINT('Ctrl Pts',(200.674069577301,29.7890397540896,29.7890397540896));
#81537=CARTESIAN_POINT('Ctrl Pts',(200.674069577301,0.,29.7890397540896));
#81538=CARTESIAN_POINT('Ctrl Pts',(200.674069577301,-29.7890397540896,29.7890397540896));
#81539=CARTESIAN_POINT('Ctrl Pts',(200.674069577301,-29.7890397540896,0.));
#81540=CARTESIAN_POINT('Ctrl Pts',(200.674069577301,-29.7890397540896,-29.7890397540896));
#81541=CARTESIAN_POINT('Ctrl Pts',(200.674069577301,0.,-29.7890397540896));
#81542=CARTESIAN_POINT('Ctrl Pts',(200.674069577301,29.7890397540896,-29.7890397540896));
#81543=CARTESIAN_POINT('Ctrl Pts',(200.674069577301,29.7890397540896,0.));
#81544=CARTESIAN_POINT('Ctrl Pts',(199.983241107359,29.9194471715901,0.));
#81545=CARTESIAN_POINT('Ctrl Pts',(199.983241107359,29.9194471715901,29.9194471715901));
#81546=CARTESIAN_POINT('Ctrl Pts',(199.983241107359,0.,29.9194471715901));
#81547=CARTESIAN_POINT('Ctrl Pts',(199.983241107359,-29.9194471715901,29.9194471715901));
#81548=CARTESIAN_POINT('Ctrl Pts',(199.983241107359,-29.9194471715901,0.));
#81549=CARTESIAN_POINT('Ctrl Pts',(199.983241107359,-29.9194471715901,-29.9194471715901));
#81550=CARTESIAN_POINT('Ctrl Pts',(199.983241107359,0.,-29.9194471715901));
#81551=CARTESIAN_POINT('Ctrl Pts',(199.983241107359,29.9194471715901,-29.9194471715901));
#81552=CARTESIAN_POINT('Ctrl Pts',(199.983241107359,29.9194471715901,0.));
#81553=CARTESIAN_POINT('Ctrl Pts',(199.279015532529,29.8458345487875,0.));
#81554=CARTESIAN_POINT('Ctrl Pts',(199.279015532529,29.8458345487875,29.8458345487875));
#81555=CARTESIAN_POINT('Ctrl Pts',(199.279015532529,0.,29.8458345487875));
#81556=CARTESIAN_POINT('Ctrl Pts',(199.279015532529,-29.8458345487875,29.8458345487875));
#81557=CARTESIAN_POINT('Ctrl Pts',(199.279015532529,-29.8458345487875,0.));
#81558=CARTESIAN_POINT('Ctrl Pts',(199.279015532529,-29.8458345487875,-29.8458345487875));
#81559=CARTESIAN_POINT('Ctrl Pts',(199.279015532529,0.,-29.8458345487875));
#81560=CARTESIAN_POINT('Ctrl Pts',(199.279015532529,29.8458345487875,-29.8458345487875));
#81561=CARTESIAN_POINT('Ctrl Pts',(199.279015532529,29.8458345487875,0.));
#81562=CARTESIAN_POINT('Ctrl Pts',(198.57393042139,29.5782809062286,0.));
#81563=CARTESIAN_POINT('Ctrl Pts',(198.57393042139,29.5782809062286,29.5782809062286));
#81564=CARTESIAN_POINT('Ctrl Pts',(198.57393042139,0.,29.5782809062286));
#81565=CARTESIAN_POINT('Ctrl Pts',(198.57393042139,-29.5782809062286,29.5782809062286));
#81566=CARTESIAN_POINT('Ctrl Pts',(198.57393042139,-29.5782809062286,0.));
#81567=CARTESIAN_POINT('Ctrl Pts',(198.57393042139,-29.5782809062286,-29.5782809062286));
#81568=CARTESIAN_POINT('Ctrl Pts',(198.57393042139,0.,-29.5782809062286));
#81569=CARTESIAN_POINT('Ctrl Pts',(198.57393042139,29.5782809062286,-29.5782809062286));
#81570=CARTESIAN_POINT('Ctrl Pts',(198.57393042139,29.5782809062286,0.));
#81571=CARTESIAN_POINT('Ctrl Pts',(197.878737400882,29.146450351934,0.));
#81572=CARTESIAN_POINT('Ctrl Pts',(197.878737400882,29.146450351934,29.146450351934));
#81573=CARTESIAN_POINT('Ctrl Pts',(197.878737400882,0.,29.146450351934));
#81574=CARTESIAN_POINT('Ctrl Pts',(197.878737400882,-29.146450351934,29.146450351934));
#81575=CARTESIAN_POINT('Ctrl Pts',(197.878737400882,-29.146450351934,0.));
#81576=CARTESIAN_POINT('Ctrl Pts',(197.878737400882,-29.146450351934,-29.146450351934));
#81577=CARTESIAN_POINT('Ctrl Pts',(197.878737400882,0.,-29.146450351934));
#81578=CARTESIAN_POINT('Ctrl Pts',(197.878737400882,29.146450351934,-29.146450351934));
#81579=CARTESIAN_POINT('Ctrl Pts',(197.878737400882,29.146450351934,0.));
#81580=CARTESIAN_POINT('Ctrl Pts',(197.201256210244,28.6080668697552,0.));
#81581=CARTESIAN_POINT('Ctrl Pts',(197.201256210244,28.6080668697552,28.6080668697552));
#81582=CARTESIAN_POINT('Ctrl Pts',(197.201256210244,0.,28.6080668697552));
#81583=CARTESIAN_POINT('Ctrl Pts',(197.201256210244,-28.6080668697552,28.6080668697552));
#81584=CARTESIAN_POINT('Ctrl Pts',(197.201256210244,-28.6080668697552,0.));
#81585=CARTESIAN_POINT('Ctrl Pts',(197.201256210244,-28.6080668697552,-28.6080668697552));
#81586=CARTESIAN_POINT('Ctrl Pts',(197.201256210244,0.,-28.6080668697552));
#81587=CARTESIAN_POINT('Ctrl Pts',(197.201256210244,28.6080668697552,-28.6080668697552));
#81588=CARTESIAN_POINT('Ctrl Pts',(197.201256210244,28.6080668697552,0.));
#81589=CARTESIAN_POINT('Ctrl Pts',(196.545471802854,28.0523886024101,0.));
#81590=CARTESIAN_POINT('Ctrl Pts',(196.545471802854,28.0523886024101,28.0523886024101));
#81591=CARTESIAN_POINT('Ctrl Pts',(196.545471802854,0.,28.0523886024101));
#81592=CARTESIAN_POINT('Ctrl Pts',(196.545471802854,-28.0523886024101,28.0523886024101));
#81593=CARTESIAN_POINT('Ctrl Pts',(196.545471802854,-28.0523886024101,0.));
#81594=CARTESIAN_POINT('Ctrl Pts',(196.545471802854,-28.0523886024101,-28.0523886024101));
#81595=CARTESIAN_POINT('Ctrl Pts',(196.545471802854,0.,-28.0523886024101));
#81596=CARTESIAN_POINT('Ctrl Pts',(196.545471802854,28.0523886024101,-28.0523886024101));
#81597=CARTESIAN_POINT('Ctrl Pts',(196.545471802854,28.0523886024101,0.));
#81598=CARTESIAN_POINT('Ctrl Pts',(195.912058185941,27.5804806183496,0.));
#81599=CARTESIAN_POINT('Ctrl Pts',(195.912058185941,27.5804806183496,27.5804806183496));
#81600=CARTESIAN_POINT('Ctrl Pts',(195.912058185941,0.,27.5804806183496));
#81601=CARTESIAN_POINT('Ctrl Pts',(195.912058185941,-27.5804806183496,27.5804806183496));
#81602=CARTESIAN_POINT('Ctrl Pts',(195.912058185941,-27.5804806183496,0.));
#81603=CARTESIAN_POINT('Ctrl Pts',(195.912058185941,-27.5804806183496,-27.5804806183496));
#81604=CARTESIAN_POINT('Ctrl Pts',(195.912058185941,0.,-27.5804806183496));
#81605=CARTESIAN_POINT('Ctrl Pts',(195.912058185941,27.5804806183496,-27.5804806183496));
#81606=CARTESIAN_POINT('Ctrl Pts',(195.912058185941,27.5804806183496,0.));
#81607=CARTESIAN_POINT('Ctrl Pts',(195.298687821752,27.2875376857686,0.));
#81608=CARTESIAN_POINT('Ctrl Pts',(195.298687821752,27.2875376857686,27.2875376857686));
#81609=CARTESIAN_POINT('Ctrl Pts',(195.298687821752,0.,27.2875376857686));
#81610=CARTESIAN_POINT('Ctrl Pts',(195.298687821752,-27.2875376857686,27.2875376857686));
#81611=CARTESIAN_POINT('Ctrl Pts',(195.298687821752,-27.2875376857686,0.));
#81612=CARTESIAN_POINT('Ctrl Pts',(195.298687821752,-27.2875376857686,-27.2875376857686));
#81613=CARTESIAN_POINT('Ctrl Pts',(195.298687821752,0.,-27.2875376857686));
#81614=CARTESIAN_POINT('Ctrl Pts',(195.298687821752,27.2875376857686,-27.2875376857686));
#81615=CARTESIAN_POINT('Ctrl Pts',(195.298687821752,27.2875376857686,0.));
#81616=CARTESIAN_POINT('Ctrl Pts',(194.700480719299,27.246160623384,0.));
#81617=CARTESIAN_POINT('Ctrl Pts',(194.700480719299,27.246160623384,27.246160623384));
#81618=CARTESIAN_POINT('Ctrl Pts',(194.700480719299,0.,27.246160623384));
#81619=CARTESIAN_POINT('Ctrl Pts',(194.700480719299,-27.246160623384,27.246160623384));
#81620=CARTESIAN_POINT('Ctrl Pts',(194.700480719299,-27.246160623384,0.));
#81621=CARTESIAN_POINT('Ctrl Pts',(194.700480719299,-27.246160623384,-27.246160623384));
#81622=CARTESIAN_POINT('Ctrl Pts',(194.700480719299,0.,-27.246160623384));
#81623=CARTESIAN_POINT('Ctrl Pts',(194.700480719299,27.246160623384,-27.246160623384));
#81624=CARTESIAN_POINT('Ctrl Pts',(194.700480719299,27.246160623384,0.));
#81625=CARTESIAN_POINT('Ctrl Pts',(194.110246528525,27.4849758320246,0.));
#81626=CARTESIAN_POINT('Ctrl Pts',(194.110246528525,27.4849758320246,27.4849758320246));
#81627=CARTESIAN_POINT('Ctrl Pts',(194.110246528525,0.,27.4849758320246));
#81628=CARTESIAN_POINT('Ctrl Pts',(194.110246528525,-27.4849758320246,27.4849758320246));
#81629=CARTESIAN_POINT('Ctrl Pts',(194.110246528525,-27.4849758320246,0.));
#81630=CARTESIAN_POINT('Ctrl Pts',(194.110246528525,-27.4849758320246,-27.4849758320246));
#81631=CARTESIAN_POINT('Ctrl Pts',(194.110246528525,0.,-27.4849758320246));
#81632=CARTESIAN_POINT('Ctrl Pts',(194.110246528525,27.4849758320246,-27.4849758320246));
#81633=CARTESIAN_POINT('Ctrl Pts',(194.110246528525,27.4849758320246,0.));
#81634=CARTESIAN_POINT('Ctrl Pts',(193.519372459537,27.9858382864175,0.));
#81635=CARTESIAN_POINT('Ctrl Pts',(193.519372459537,27.9858382864175,27.9858382864175));
#81636=CARTESIAN_POINT('Ctrl Pts',(193.519372459537,0.,27.9858382864175));
#81637=CARTESIAN_POINT('Ctrl Pts',(193.519372459537,-27.9858382864175,27.9858382864175));
#81638=CARTESIAN_POINT('Ctrl Pts',(193.519372459537,-27.9858382864175,0.));
#81639=CARTESIAN_POINT('Ctrl Pts',(193.519372459537,-27.9858382864175,-27.9858382864175));
#81640=CARTESIAN_POINT('Ctrl Pts',(193.519372459537,0.,-27.9858382864175));
#81641=CARTESIAN_POINT('Ctrl Pts',(193.519372459537,27.9858382864175,-27.9858382864175));
#81642=CARTESIAN_POINT('Ctrl Pts',(193.519372459537,27.9858382864175,0.));
#81643=CARTESIAN_POINT('Ctrl Pts',(192.919287538658,28.6998106357671,0.));
#81644=CARTESIAN_POINT('Ctrl Pts',(192.919287538658,28.6998106357671,28.6998106357671));
#81645=CARTESIAN_POINT('Ctrl Pts',(192.919287538658,0.,28.6998106357671));
#81646=CARTESIAN_POINT('Ctrl Pts',(192.919287538658,-28.6998106357671,28.6998106357671));
#81647=CARTESIAN_POINT('Ctrl Pts',(192.919287538658,-28.6998106357671,0.));
#81648=CARTESIAN_POINT('Ctrl Pts',(192.919287538658,-28.6998106357671,-28.6998106357671));
#81649=CARTESIAN_POINT('Ctrl Pts',(192.919287538658,0.,-28.6998106357671));
#81650=CARTESIAN_POINT('Ctrl Pts',(192.919287538658,28.6998106357671,-28.6998106357671));
#81651=CARTESIAN_POINT('Ctrl Pts',(192.919287538658,28.6998106357671,0.));
#81652=CARTESIAN_POINT('Ctrl Pts',(192.302852321524,29.5583582075276,0.));
#81653=CARTESIAN_POINT('Ctrl Pts',(192.302852321524,29.5583582075276,29.5583582075276));
#81654=CARTESIAN_POINT('Ctrl Pts',(192.302852321524,0.,29.5583582075276));
#81655=CARTESIAN_POINT('Ctrl Pts',(192.302852321524,-29.5583582075276,29.5583582075276));
#81656=CARTESIAN_POINT('Ctrl Pts',(192.302852321524,-29.5583582075276,0.));
#81657=CARTESIAN_POINT('Ctrl Pts',(192.302852321524,-29.5583582075276,-29.5583582075276));
#81658=CARTESIAN_POINT('Ctrl Pts',(192.302852321524,0.,-29.5583582075276));
#81659=CARTESIAN_POINT('Ctrl Pts',(192.302852321524,29.5583582075276,-29.5583582075276));
#81660=CARTESIAN_POINT('Ctrl Pts',(192.302852321524,29.5583582075276,0.));
#81661=CARTESIAN_POINT('Ctrl Pts',(191.665604121366,30.4857275954352,0.));
#81662=CARTESIAN_POINT('Ctrl Pts',(191.665604121366,30.4857275954352,30.4857275954352));
#81663=CARTESIAN_POINT('Ctrl Pts',(191.665604121366,0.,30.4857275954352));
#81664=CARTESIAN_POINT('Ctrl Pts',(191.665604121366,-30.4857275954352,30.4857275954352));
#81665=CARTESIAN_POINT('Ctrl Pts',(191.665604121366,-30.4857275954352,0.));
#81666=CARTESIAN_POINT('Ctrl Pts',(191.665604121366,-30.4857275954352,-30.4857275954352));
#81667=CARTESIAN_POINT('Ctrl Pts',(191.665604121366,0.,-30.4857275954352));
#81668=CARTESIAN_POINT('Ctrl Pts',(191.665604121366,30.4857275954352,-30.4857275954352));
#81669=CARTESIAN_POINT('Ctrl Pts',(191.665604121366,30.4857275954352,0.));
#81670=CARTESIAN_POINT('Ctrl Pts',(191.007499403008,31.4126397968556,0.));
#81671=CARTESIAN_POINT('Ctrl Pts',(191.007499403008,31.4126397968556,31.4126397968556));
#81672=CARTESIAN_POINT('Ctrl Pts',(191.007499403008,0.,31.4126397968556));
#81673=CARTESIAN_POINT('Ctrl Pts',(191.007499403008,-31.4126397968556,31.4126397968556));
#81674=CARTESIAN_POINT('Ctrl Pts',(191.007499403008,-31.4126397968556,0.));
#81675=CARTESIAN_POINT('Ctrl Pts',(191.007499403008,-31.4126397968556,-31.4126397968556));
#81676=CARTESIAN_POINT('Ctrl Pts',(191.007499403008,0.,-31.4126397968556));
#81677=CARTESIAN_POINT('Ctrl Pts',(191.007499403008,31.4126397968556,-31.4126397968556));
#81678=CARTESIAN_POINT('Ctrl Pts',(191.007499403008,31.4126397968556,0.));
#81679=CARTESIAN_POINT('Ctrl Pts',(190.332663752398,32.2818828529496,0.));
#81680=CARTESIAN_POINT('Ctrl Pts',(190.332663752398,32.2818828529496,32.2818828529496));
#81681=CARTESIAN_POINT('Ctrl Pts',(190.332663752398,0.,32.2818828529496));
#81682=CARTESIAN_POINT('Ctrl Pts',(190.332663752398,-32.2818828529496,32.2818828529496));
#81683=CARTESIAN_POINT('Ctrl Pts',(190.332663752398,-32.2818828529496,0.));
#81684=CARTESIAN_POINT('Ctrl Pts',(190.332663752398,-32.2818828529496,-32.2818828529496));
#81685=CARTESIAN_POINT('Ctrl Pts',(190.332663752398,0.,-32.2818828529496));
#81686=CARTESIAN_POINT('Ctrl Pts',(190.332663752398,32.2818828529496,-32.2818828529496));
#81687=CARTESIAN_POINT('Ctrl Pts',(190.332663752398,32.2818828529496,0.));
#81688=CARTESIAN_POINT('Ctrl Pts',(189.647329687564,33.0461922340397,0.));
#81689=CARTESIAN_POINT('Ctrl Pts',(189.647329687564,33.0461922340397,33.0461922340397));
#81690=CARTESIAN_POINT('Ctrl Pts',(189.647329687564,0.,33.0461922340397));
#81691=CARTESIAN_POINT('Ctrl Pts',(189.647329687564,-33.0461922340397,33.0461922340397));
#81692=CARTESIAN_POINT('Ctrl Pts',(189.647329687564,-33.0461922340397,0.));
#81693=CARTESIAN_POINT('Ctrl Pts',(189.647329687564,-33.0461922340397,-33.0461922340397));
#81694=CARTESIAN_POINT('Ctrl Pts',(189.647329687564,0.,-33.0461922340397));
#81695=CARTESIAN_POINT('Ctrl Pts',(189.647329687564,33.0461922340397,-33.0461922340397));
#81696=CARTESIAN_POINT('Ctrl Pts',(189.647329687564,33.0461922340397,0.));
#81697=CARTESIAN_POINT('Ctrl Pts',(188.958330678398,33.6683706359231,0.));
#81698=CARTESIAN_POINT('Ctrl Pts',(188.958330678398,33.6683706359231,33.6683706359231));
#81699=CARTESIAN_POINT('Ctrl Pts',(188.958330678398,0.,33.6683706359231));
#81700=CARTESIAN_POINT('Ctrl Pts',(188.958330678398,-33.6683706359231,33.6683706359231));
#81701=CARTESIAN_POINT('Ctrl Pts',(188.958330678398,-33.6683706359231,0.));
#81702=CARTESIAN_POINT('Ctrl Pts',(188.958330678398,-33.6683706359231,-33.6683706359231));
#81703=CARTESIAN_POINT('Ctrl Pts',(188.958330678398,0.,-33.6683706359231));
#81704=CARTESIAN_POINT('Ctrl Pts',(188.958330678398,33.6683706359231,-33.6683706359231));
#81705=CARTESIAN_POINT('Ctrl Pts',(188.958330678398,33.6683706359231,0.));
#81706=CARTESIAN_POINT('Ctrl Pts',(188.271268152939,34.1203973311724,0.));
#81707=CARTESIAN_POINT('Ctrl Pts',(188.271268152939,34.1203973311724,34.1203973311724));
#81708=CARTESIAN_POINT('Ctrl Pts',(188.271268152939,0.,34.1203973311724));
#81709=CARTESIAN_POINT('Ctrl Pts',(188.271268152939,-34.1203973311724,34.1203973311724));
#81710=CARTESIAN_POINT('Ctrl Pts',(188.271268152939,-34.1203973311724,0.));
#81711=CARTESIAN_POINT('Ctrl Pts',(188.271268152939,-34.1203973311724,-34.1203973311724));
#81712=CARTESIAN_POINT('Ctrl Pts',(188.271268152939,0.,-34.1203973311724));
#81713=CARTESIAN_POINT('Ctrl Pts',(188.271268152939,34.1203973311724,-34.1203973311724));
#81714=CARTESIAN_POINT('Ctrl Pts',(188.271268152939,34.1203973311724,0.));
#81715=CARTESIAN_POINT('Ctrl Pts',(187.589050043455,34.3832180811066,0.));
#81716=CARTESIAN_POINT('Ctrl Pts',(187.589050043455,34.3832180811066,34.3832180811066));
#81717=CARTESIAN_POINT('Ctrl Pts',(187.589050043455,0.,34.3832180811066));
#81718=CARTESIAN_POINT('Ctrl Pts',(187.589050043455,-34.3832180811066,34.3832180811066));
#81719=CARTESIAN_POINT('Ctrl Pts',(187.589050043455,-34.3832180811066,0.));
#81720=CARTESIAN_POINT('Ctrl Pts',(187.589050043455,-34.3832180811066,-34.3832180811066));
#81721=CARTESIAN_POINT('Ctrl Pts',(187.589050043455,0.,-34.3832180811066));
#81722=CARTESIAN_POINT('Ctrl Pts',(187.589050043455,34.3832180811066,-34.3832180811066));
#81723=CARTESIAN_POINT('Ctrl Pts',(187.589050043455,34.3832180811066,0.));
#81724=CARTESIAN_POINT('Ctrl Pts',(186.909683874378,34.4456555286542,0.));
#81725=CARTESIAN_POINT('Ctrl Pts',(186.909683874378,34.4456555286541,34.4456555286541));
#81726=CARTESIAN_POINT('Ctrl Pts',(186.909683874378,0.,34.4456555286542));
#81727=CARTESIAN_POINT('Ctrl Pts',(186.909683874378,-34.4456555286541,34.4456555286541));
#81728=CARTESIAN_POINT('Ctrl Pts',(186.909683874378,-34.4456555286542,0.));
#81729=CARTESIAN_POINT('Ctrl Pts',(186.909683874378,-34.4456555286541,-34.4456555286541));
#81730=CARTESIAN_POINT('Ctrl Pts',(186.909683874378,0.,-34.4456555286542));
#81731=CARTESIAN_POINT('Ctrl Pts',(186.909683874378,34.4456555286541,-34.4456555286541));
#81732=CARTESIAN_POINT('Ctrl Pts',(186.909683874378,34.4456555286542,0.));
#81733=CARTESIAN_POINT('Ctrl Pts',(186.227093638197,34.3065527505812,0.));
#81734=CARTESIAN_POINT('Ctrl Pts',(186.227093638197,34.3065527505812,34.3065527505812));
#81735=CARTESIAN_POINT('Ctrl Pts',(186.227093638197,0.,34.3065527505812));
#81736=CARTESIAN_POINT('Ctrl Pts',(186.227093638197,-34.3065527505812,34.3065527505812));
#81737=CARTESIAN_POINT('Ctrl Pts',(186.227093638197,-34.3065527505812,0.));
#81738=CARTESIAN_POINT('Ctrl Pts',(186.227093638197,-34.3065527505812,-34.3065527505812));
#81739=CARTESIAN_POINT('Ctrl Pts',(186.227093638197,0.,-34.3065527505812));
#81740=CARTESIAN_POINT('Ctrl Pts',(186.227093638197,34.3065527505812,-34.3065527505812));
#81741=CARTESIAN_POINT('Ctrl Pts',(186.227093638197,34.3065527505812,0.));
#81742=CARTESIAN_POINT('Ctrl Pts',(185.533966240925,33.9792969407959,0.));
#81743=CARTESIAN_POINT('Ctrl Pts',(185.533966240925,33.9792969407959,33.9792969407959));
#81744=CARTESIAN_POINT('Ctrl Pts',(185.533966240925,0.,33.9792969407959));
#81745=CARTESIAN_POINT('Ctrl Pts',(185.533966240925,-33.9792969407959,33.9792969407959));
#81746=CARTESIAN_POINT('Ctrl Pts',(185.533966240925,-33.9792969407959,0.));
#81747=CARTESIAN_POINT('Ctrl Pts',(185.533966240925,-33.9792969407959,-33.9792969407959));
#81748=CARTESIAN_POINT('Ctrl Pts',(185.533966240925,0.,-33.9792969407959));
#81749=CARTESIAN_POINT('Ctrl Pts',(185.533966240925,33.9792969407959,-33.9792969407959));
#81750=CARTESIAN_POINT('Ctrl Pts',(185.533966240925,33.9792969407959,0.));
#81751=CARTESIAN_POINT('Ctrl Pts',(184.823852750706,33.4950850843424,0.));
#81752=CARTESIAN_POINT('Ctrl Pts',(184.823852750706,33.4950850843424,33.4950850843424));
#81753=CARTESIAN_POINT('Ctrl Pts',(184.823852750706,0.,33.4950850843424));
#81754=CARTESIAN_POINT('Ctrl Pts',(184.823852750706,-33.4950850843424,33.4950850843424));
#81755=CARTESIAN_POINT('Ctrl Pts',(184.823852750706,-33.4950850843424,0.));
#81756=CARTESIAN_POINT('Ctrl Pts',(184.823852750706,-33.4950850843424,-33.4950850843424));
#81757=CARTESIAN_POINT('Ctrl Pts',(184.823852750706,0.,-33.4950850843424));
#81758=CARTESIAN_POINT('Ctrl Pts',(184.823852750706,33.4950850843424,-33.4950850843424));
#81759=CARTESIAN_POINT('Ctrl Pts',(184.823852750706,33.4950850843424,0.));
#81760=CARTESIAN_POINT('Ctrl Pts',(184.093886879022,32.9080070117905,0.));
#81761=CARTESIAN_POINT('Ctrl Pts',(184.093886879022,32.9080070117905,32.9080070117905));
#81762=CARTESIAN_POINT('Ctrl Pts',(184.093886879022,0.,32.9080070117905));
#81763=CARTESIAN_POINT('Ctrl Pts',(184.093886879022,-32.9080070117905,32.9080070117905));
#81764=CARTESIAN_POINT('Ctrl Pts',(184.093886879022,-32.9080070117905,0.));
#81765=CARTESIAN_POINT('Ctrl Pts',(184.093886879022,-32.9080070117905,-32.9080070117905));
#81766=CARTESIAN_POINT('Ctrl Pts',(184.093886879022,0.,-32.9080070117905));
#81767=CARTESIAN_POINT('Ctrl Pts',(184.093886879022,32.9080070117905,-32.9080070117905));
#81768=CARTESIAN_POINT('Ctrl Pts',(184.093886879022,32.9080070117905,0.));
#81769=CARTESIAN_POINT('Ctrl Pts',(183.346276790563,32.2953778251868,0.));
#81770=CARTESIAN_POINT('Ctrl Pts',(183.346276790563,32.2953778251867,32.2953778251867));
#81771=CARTESIAN_POINT('Ctrl Pts',(183.346276790563,0.,32.2953778251868));
#81772=CARTESIAN_POINT('Ctrl Pts',(183.346276790563,-32.2953778251867,32.2953778251867));
#81773=CARTESIAN_POINT('Ctrl Pts',(183.346276790563,-32.2953778251868,0.));
#81774=CARTESIAN_POINT('Ctrl Pts',(183.346276790563,-32.2953778251867,-32.2953778251867));
#81775=CARTESIAN_POINT('Ctrl Pts',(183.346276790563,0.,-32.2953778251868));
#81776=CARTESIAN_POINT('Ctrl Pts',(183.346276790563,32.2953778251867,-32.2953778251867));
#81777=CARTESIAN_POINT('Ctrl Pts',(183.346276790563,32.2953778251868,0.));
#81778=CARTESIAN_POINT('Ctrl Pts',(182.586327425199,31.7435152517629,0.));
#81779=CARTESIAN_POINT('Ctrl Pts',(182.586327425199,31.7435152517629,31.7435152517629));
#81780=CARTESIAN_POINT('Ctrl Pts',(182.586327425199,0.,31.7435152517629));
#81781=CARTESIAN_POINT('Ctrl Pts',(182.586327425199,-31.7435152517629,31.7435152517629));
#81782=CARTESIAN_POINT('Ctrl Pts',(182.586327425199,-31.7435152517629,0.));
#81783=CARTESIAN_POINT('Ctrl Pts',(182.586327425199,-31.7435152517629,-31.7435152517629));
#81784=CARTESIAN_POINT('Ctrl Pts',(182.586327425199,0.,-31.7435152517629));
#81785=CARTESIAN_POINT('Ctrl Pts',(182.586327425199,31.7435152517629,-31.7435152517629));
#81786=CARTESIAN_POINT('Ctrl Pts',(182.586327425199,31.7435152517629,0.));
#81787=CARTESIAN_POINT('Ctrl Pts',(181.821060794834,31.336111008946,0.));
#81788=CARTESIAN_POINT('Ctrl Pts',(181.821060794834,31.336111008946,31.336111008946));
#81789=CARTESIAN_POINT('Ctrl Pts',(181.821060794834,0.,31.336111008946));
#81790=CARTESIAN_POINT('Ctrl Pts',(181.821060794834,-31.336111008946,31.336111008946));
#81791=CARTESIAN_POINT('Ctrl Pts',(181.821060794834,-31.336111008946,0.));
#81792=CARTESIAN_POINT('Ctrl Pts',(181.821060794834,-31.336111008946,-31.336111008946));
#81793=CARTESIAN_POINT('Ctrl Pts',(181.821060794834,0.,-31.336111008946));
#81794=CARTESIAN_POINT('Ctrl Pts',(181.821060794834,31.336111008946,-31.336111008946));
#81795=CARTESIAN_POINT('Ctrl Pts',(181.821060794834,31.336111008946,0.));
#81796=CARTESIAN_POINT('Ctrl Pts',(181.057582682021,31.141384874781,0.));
#81797=CARTESIAN_POINT('Ctrl Pts',(181.057582682021,31.141384874781,31.141384874781));
#81798=CARTESIAN_POINT('Ctrl Pts',(181.057582682021,0.,31.141384874781));
#81799=CARTESIAN_POINT('Ctrl Pts',(181.057582682021,-31.141384874781,31.141384874781));
#81800=CARTESIAN_POINT('Ctrl Pts',(181.057582682021,-31.141384874781,0.));
#81801=CARTESIAN_POINT('Ctrl Pts',(181.057582682021,-31.141384874781,-31.141384874781));
#81802=CARTESIAN_POINT('Ctrl Pts',(181.057582682021,0.,-31.141384874781));
#81803=CARTESIAN_POINT('Ctrl Pts',(181.057582682021,31.141384874781,-31.141384874781));
#81804=CARTESIAN_POINT('Ctrl Pts',(181.057582682021,31.141384874781,0.));
#81805=CARTESIAN_POINT('Ctrl Pts',(180.301606849543,31.2002008326786,0.));
#81806=CARTESIAN_POINT('Ctrl Pts',(180.301606849543,31.2002008326786,31.2002008326786));
#81807=CARTESIAN_POINT('Ctrl Pts',(180.301606849543,0.,31.2002008326786));
#81808=CARTESIAN_POINT('Ctrl Pts',(180.301606849543,-31.2002008326786,31.2002008326786));
#81809=CARTESIAN_POINT('Ctrl Pts',(180.301606849543,-31.2002008326786,0.));
#81810=CARTESIAN_POINT('Ctrl Pts',(180.301606849543,-31.2002008326786,-31.2002008326786));
#81811=CARTESIAN_POINT('Ctrl Pts',(180.301606849543,0.,-31.2002008326786));
#81812=CARTESIAN_POINT('Ctrl Pts',(180.301606849543,31.2002008326786,-31.2002008326786));
#81813=CARTESIAN_POINT('Ctrl Pts',(180.301606849543,31.2002008326786,0.));
#81814=CARTESIAN_POINT('Ctrl Pts',(179.555779619084,31.5125164881584,0.));
#81815=CARTESIAN_POINT('Ctrl Pts',(179.555779619084,31.5125164881584,31.5125164881584));
#81816=CARTESIAN_POINT('Ctrl Pts',(179.555779619084,0.,31.5125164881584));
#81817=CARTESIAN_POINT('Ctrl Pts',(179.555779619084,-31.5125164881584,31.5125164881584));
#81818=CARTESIAN_POINT('Ctrl Pts',(179.555779619084,-31.5125164881584,0.));
#81819=CARTESIAN_POINT('Ctrl Pts',(179.555779619084,-31.5125164881584,-31.5125164881584));
#81820=CARTESIAN_POINT('Ctrl Pts',(179.555779619084,0.,-31.5125164881584));
#81821=CARTESIAN_POINT('Ctrl Pts',(179.555779619084,31.5125164881584,-31.5125164881584));
#81822=CARTESIAN_POINT('Ctrl Pts',(179.555779619084,31.5125164881584,0.));
#81823=CARTESIAN_POINT('Ctrl Pts',(178.82040630265,32.0463508095147,0.));
#81824=CARTESIAN_POINT('Ctrl Pts',(178.82040630265,32.0463508095147,32.0463508095147));
#81825=CARTESIAN_POINT('Ctrl Pts',(178.82040630265,0.,32.0463508095147));
#81826=CARTESIAN_POINT('Ctrl Pts',(178.82040630265,-32.0463508095147,32.0463508095147));
#81827=CARTESIAN_POINT('Ctrl Pts',(178.82040630265,-32.0463508095147,0.));
#81828=CARTESIAN_POINT('Ctrl Pts',(178.82040630265,-32.0463508095147,-32.0463508095147));
#81829=CARTESIAN_POINT('Ctrl Pts',(178.82040630265,0.,-32.0463508095147));
#81830=CARTESIAN_POINT('Ctrl Pts',(178.82040630265,32.0463508095147,-32.0463508095147));
#81831=CARTESIAN_POINT('Ctrl Pts',(178.82040630265,32.0463508095147,0.));
#81832=CARTESIAN_POINT('Ctrl Pts',(178.094333722328,32.7483045448037,0.));
#81833=CARTESIAN_POINT('Ctrl Pts',(178.094333722328,32.7483045448037,32.7483045448037));
#81834=CARTESIAN_POINT('Ctrl Pts',(178.094333722328,0.,32.7483045448037));
#81835=CARTESIAN_POINT('Ctrl Pts',(178.094333722328,-32.7483045448037,32.7483045448037));
#81836=CARTESIAN_POINT('Ctrl Pts',(178.094333722328,-32.7483045448037,0.));
#81837=CARTESIAN_POINT('Ctrl Pts',(178.094333722328,-32.7483045448037,-32.7483045448037));
#81838=CARTESIAN_POINT('Ctrl Pts',(178.094333722328,0.,-32.7483045448037));
#81839=CARTESIAN_POINT('Ctrl Pts',(178.094333722328,32.7483045448037,-32.7483045448037));
#81840=CARTESIAN_POINT('Ctrl Pts',(178.094333722328,32.7483045448037,0.));
#81841=CARTESIAN_POINT('Ctrl Pts',(177.375813082222,33.5537582813009,0.));
#81842=CARTESIAN_POINT('Ctrl Pts',(177.375813082222,33.5537582813009,33.5537582813009));
#81843=CARTESIAN_POINT('Ctrl Pts',(177.375813082222,0.,33.5537582813009));
#81844=CARTESIAN_POINT('Ctrl Pts',(177.375813082222,-33.5537582813009,33.5537582813009));
#81845=CARTESIAN_POINT('Ctrl Pts',(177.375813082222,-33.5537582813009,0.));
#81846=CARTESIAN_POINT('Ctrl Pts',(177.375813082222,-33.5537582813009,-33.5537582813009));
#81847=CARTESIAN_POINT('Ctrl Pts',(177.375813082222,0.,-33.5537582813009));
#81848=CARTESIAN_POINT('Ctrl Pts',(177.375813082222,33.5537582813009,-33.5537582813009));
#81849=CARTESIAN_POINT('Ctrl Pts',(177.375813082222,33.5537582813009,0.));
#81850=CARTESIAN_POINT('Ctrl Pts',(176.663284323105,34.3965983321123,0.));
#81851=CARTESIAN_POINT('Ctrl Pts',(176.663284323105,34.3965983321123,34.3965983321123));
#81852=CARTESIAN_POINT('Ctrl Pts',(176.663284323105,0.,34.3965983321123));
#81853=CARTESIAN_POINT('Ctrl Pts',(176.663284323105,-34.3965983321123,34.3965983321123));
#81854=CARTESIAN_POINT('Ctrl Pts',(176.663284323105,-34.3965983321123,0.));
#81855=CARTESIAN_POINT('Ctrl Pts',(176.663284323105,-34.3965983321123,-34.3965983321123));
#81856=CARTESIAN_POINT('Ctrl Pts',(176.663284323105,0.,-34.3965983321123));
#81857=CARTESIAN_POINT('Ctrl Pts',(176.663284323105,34.3965983321123,-34.3965983321123));
#81858=CARTESIAN_POINT('Ctrl Pts',(176.663284323105,34.3965983321123,0.));
#81859=CARTESIAN_POINT('Ctrl Pts',(175.956404761947,35.220592169579,0.));
#81860=CARTESIAN_POINT('Ctrl Pts',(175.956404761947,35.220592169579,35.220592169579));
#81861=CARTESIAN_POINT('Ctrl Pts',(175.956404761947,0.,35.220592169579));
#81862=CARTESIAN_POINT('Ctrl Pts',(175.956404761947,-35.220592169579,35.220592169579));
#81863=CARTESIAN_POINT('Ctrl Pts',(175.956404761947,-35.220592169579,0.));
#81864=CARTESIAN_POINT('Ctrl Pts',(175.956404761947,-35.220592169579,-35.220592169579));
#81865=CARTESIAN_POINT('Ctrl Pts',(175.956404761947,0.,-35.220592169579));
#81866=CARTESIAN_POINT('Ctrl Pts',(175.956404761947,35.220592169579,-35.220592169579));
#81867=CARTESIAN_POINT('Ctrl Pts',(175.956404761947,35.220592169579,0.));
#81868=CARTESIAN_POINT('Ctrl Pts',(175.256166976199,35.9845194006668,0.));
#81869=CARTESIAN_POINT('Ctrl Pts',(175.256166976199,35.9845194006668,35.9845194006668));
#81870=CARTESIAN_POINT('Ctrl Pts',(175.256166976199,0.,35.9845194006668));
#81871=CARTESIAN_POINT('Ctrl Pts',(175.256166976199,-35.9845194006668,35.9845194006668));
#81872=CARTESIAN_POINT('Ctrl Pts',(175.256166976199,-35.9845194006668,0.));
#81873=CARTESIAN_POINT('Ctrl Pts',(175.256166976199,-35.9845194006668,-35.9845194006668));
#81874=CARTESIAN_POINT('Ctrl Pts',(175.256166976199,0.,-35.9845194006668));
#81875=CARTESIAN_POINT('Ctrl Pts',(175.256166976199,35.9845194006668,-35.9845194006668));
#81876=CARTESIAN_POINT('Ctrl Pts',(175.256166976199,35.9845194006668,0.));
#81877=CARTESIAN_POINT('Ctrl Pts',(174.563968613803,36.6602217315156,0.));
#81878=CARTESIAN_POINT('Ctrl Pts',(174.563968613803,36.6602217315156,36.6602217315156));
#81879=CARTESIAN_POINT('Ctrl Pts',(174.563968613803,0.,36.6602217315156));
#81880=CARTESIAN_POINT('Ctrl Pts',(174.563968613803,-36.6602217315156,36.6602217315156));
#81881=CARTESIAN_POINT('Ctrl Pts',(174.563968613803,-36.6602217315156,0.));
#81882=CARTESIAN_POINT('Ctrl Pts',(174.563968613803,-36.6602217315156,-36.6602217315156));
#81883=CARTESIAN_POINT('Ctrl Pts',(174.563968613803,0.,-36.6602217315156));
#81884=CARTESIAN_POINT('Ctrl Pts',(174.563968613803,36.6602217315156,-36.6602217315156));
#81885=CARTESIAN_POINT('Ctrl Pts',(174.563968613803,36.6602217315156,0.));
#81886=CARTESIAN_POINT('Ctrl Pts',(173.88097676403,37.2324839644745,0.));
#81887=CARTESIAN_POINT('Ctrl Pts',(173.88097676403,37.2324839644744,37.2324839644744));
#81888=CARTESIAN_POINT('Ctrl Pts',(173.88097676403,0.,37.2324839644745));
#81889=CARTESIAN_POINT('Ctrl Pts',(173.88097676403,-37.2324839644744,37.2324839644744));
#81890=CARTESIAN_POINT('Ctrl Pts',(173.88097676403,-37.2324839644745,0.));
#81891=CARTESIAN_POINT('Ctrl Pts',(173.88097676403,-37.2324839644744,-37.2324839644744));
#81892=CARTESIAN_POINT('Ctrl Pts',(173.88097676403,0.,-37.2324839644745));
#81893=CARTESIAN_POINT('Ctrl Pts',(173.88097676403,37.2324839644744,-37.2324839644744));
#81894=CARTESIAN_POINT('Ctrl Pts',(173.88097676403,37.2324839644745,0.));
#81895=CARTESIAN_POINT('Ctrl Pts',(173.207330843265,37.6982699366733,0.));
#81896=CARTESIAN_POINT('Ctrl Pts',(173.207330843265,37.6982699366733,37.6982699366733));
#81897=CARTESIAN_POINT('Ctrl Pts',(173.207330843265,0.,37.6982699366733));
#81898=CARTESIAN_POINT('Ctrl Pts',(173.207330843265,-37.6982699366733,37.6982699366733));
#81899=CARTESIAN_POINT('Ctrl Pts',(173.207330843265,-37.6982699366733,0.));
#81900=CARTESIAN_POINT('Ctrl Pts',(173.207330843265,-37.6982699366733,-37.6982699366733));
#81901=CARTESIAN_POINT('Ctrl Pts',(173.207330843265,0.,-37.6982699366733));
#81902=CARTESIAN_POINT('Ctrl Pts',(173.207330843265,37.6982699366733,-37.6982699366733));
#81903=CARTESIAN_POINT('Ctrl Pts',(173.207330843265,37.6982699366733,0.));
#81904=CARTESIAN_POINT('Ctrl Pts',(172.541509808549,38.0660475925471,0.));
#81905=CARTESIAN_POINT('Ctrl Pts',(172.541509808549,38.0660475925471,38.0660475925471));
#81906=CARTESIAN_POINT('Ctrl Pts',(172.541509808549,0.,38.0660475925471));
#81907=CARTESIAN_POINT('Ctrl Pts',(172.541509808549,-38.0660475925471,38.0660475925471));
#81908=CARTESIAN_POINT('Ctrl Pts',(172.541509808549,-38.0660475925471,0.));
#81909=CARTESIAN_POINT('Ctrl Pts',(172.541509808549,-38.0660475925471,-38.0660475925471));
#81910=CARTESIAN_POINT('Ctrl Pts',(172.541509808549,0.,-38.0660475925471));
#81911=CARTESIAN_POINT('Ctrl Pts',(172.541509808549,38.0660475925471,-38.0660475925471));
#81912=CARTESIAN_POINT('Ctrl Pts',(172.541509808549,38.0660475925471,0.));
#81913=CARTESIAN_POINT('Ctrl Pts',(171.879381987014,38.35560208533,0.));
#81914=CARTESIAN_POINT('Ctrl Pts',(171.879381987014,38.35560208533,38.35560208533));
#81915=CARTESIAN_POINT('Ctrl Pts',(171.879381987014,0.,38.35560208533));
#81916=CARTESIAN_POINT('Ctrl Pts',(171.879381987014,-38.35560208533,38.35560208533));
#81917=CARTESIAN_POINT('Ctrl Pts',(171.879381987014,-38.35560208533,0.));
#81918=CARTESIAN_POINT('Ctrl Pts',(171.879381987014,-38.35560208533,-38.35560208533));
#81919=CARTESIAN_POINT('Ctrl Pts',(171.879381987014,0.,-38.35560208533));
#81920=CARTESIAN_POINT('Ctrl Pts',(171.879381987014,38.35560208533,-38.35560208533));
#81921=CARTESIAN_POINT('Ctrl Pts',(171.879381987014,38.35560208533,0.));
#81922=CARTESIAN_POINT('Ctrl Pts',(171.214744140827,38.5947917128636,0.));
#81923=CARTESIAN_POINT('Ctrl Pts',(171.214744140827,38.5947917128636,38.5947917128636));
#81924=CARTESIAN_POINT('Ctrl Pts',(171.214744140827,0.,38.5947917128636));
#81925=CARTESIAN_POINT('Ctrl Pts',(171.214744140827,-38.5947917128636,38.5947917128636));
#81926=CARTESIAN_POINT('Ctrl Pts',(171.214744140827,-38.5947917128636,0.));
#81927=CARTESIAN_POINT('Ctrl Pts',(171.214744140827,-38.5947917128636,-38.5947917128636));
#81928=CARTESIAN_POINT('Ctrl Pts',(171.214744140827,0.,-38.5947917128636));
#81929=CARTESIAN_POINT('Ctrl Pts',(171.214744140827,38.5947917128636,-38.5947917128636));
#81930=CARTESIAN_POINT('Ctrl Pts',(171.214744140827,38.5947917128636,0.));
#81931=CARTESIAN_POINT('Ctrl Pts',(170.540530769115,38.8148056986339,0.));
#81932=CARTESIAN_POINT('Ctrl Pts',(170.540530769115,38.8148056986339,38.8148056986339));
#81933=CARTESIAN_POINT('Ctrl Pts',(170.540530769115,0.,38.8148056986339));
#81934=CARTESIAN_POINT('Ctrl Pts',(170.540530769115,-38.8148056986339,38.8148056986339));
#81935=CARTESIAN_POINT('Ctrl Pts',(170.540530769115,-38.8148056986339,0.));
#81936=CARTESIAN_POINT('Ctrl Pts',(170.540530769115,-38.8148056986339,-38.8148056986339));
#81937=CARTESIAN_POINT('Ctrl Pts',(170.540530769115,0.,-38.8148056986339));
#81938=CARTESIAN_POINT('Ctrl Pts',(170.540530769115,38.8148056986339,-38.8148056986339));
#81939=CARTESIAN_POINT('Ctrl Pts',(170.540530769115,38.8148056986339,0.));
#81940=CARTESIAN_POINT('Ctrl Pts',(169.849764887444,39.0460911245127,0.));
#81941=CARTESIAN_POINT('Ctrl Pts',(169.849764887444,39.0460911245127,39.0460911245127));
#81942=CARTESIAN_POINT('Ctrl Pts',(169.849764887444,0.,39.0460911245127));
#81943=CARTESIAN_POINT('Ctrl Pts',(169.849764887444,-39.0460911245127,39.0460911245127));
#81944=CARTESIAN_POINT('Ctrl Pts',(169.849764887444,-39.0460911245127,0.));
#81945=CARTESIAN_POINT('Ctrl Pts',(169.849764887444,-39.0460911245127,-39.0460911245127));
#81946=CARTESIAN_POINT('Ctrl Pts',(169.849764887444,0.,-39.0460911245127));
#81947=CARTESIAN_POINT('Ctrl Pts',(169.849764887444,39.0460911245127,-39.0460911245127));
#81948=CARTESIAN_POINT('Ctrl Pts',(169.849764887444,39.0460911245127,0.));
#81949=CARTESIAN_POINT('Ctrl Pts',(169.136715408109,39.3135851151319,0.));
#81950=CARTESIAN_POINT('Ctrl Pts',(169.136715408109,39.3135851151319,39.3135851151319));
#81951=CARTESIAN_POINT('Ctrl Pts',(169.136715408109,0.,39.3135851151319));
#81952=CARTESIAN_POINT('Ctrl Pts',(169.136715408109,-39.3135851151319,39.3135851151319));
#81953=CARTESIAN_POINT('Ctrl Pts',(169.136715408109,-39.3135851151319,0.));
#81954=CARTESIAN_POINT('Ctrl Pts',(169.136715408109,-39.3135851151319,-39.3135851151319));
#81955=CARTESIAN_POINT('Ctrl Pts',(169.136715408109,0.,-39.3135851151319));
#81956=CARTESIAN_POINT('Ctrl Pts',(169.136715408109,39.3135851151319,-39.3135851151319));
#81957=CARTESIAN_POINT('Ctrl Pts',(169.136715408109,39.3135851151319,0.));
#81958=CARTESIAN_POINT('Ctrl Pts',(168.397662779334,39.63351813324,0.));
#81959=CARTESIAN_POINT('Ctrl Pts',(168.397662779334,39.63351813324,39.63351813324));
#81960=CARTESIAN_POINT('Ctrl Pts',(168.397662779334,0.,39.63351813324));
#81961=CARTESIAN_POINT('Ctrl Pts',(168.397662779334,-39.63351813324,39.63351813324));
#81962=CARTESIAN_POINT('Ctrl Pts',(168.397662779334,-39.63351813324,0.));
#81963=CARTESIAN_POINT('Ctrl Pts',(168.397662779334,-39.63351813324,-39.63351813324));
#81964=CARTESIAN_POINT('Ctrl Pts',(168.397662779334,0.,-39.63351813324));
#81965=CARTESIAN_POINT('Ctrl Pts',(168.397662779334,39.63351813324,-39.63351813324));
#81966=CARTESIAN_POINT('Ctrl Pts',(168.397662779334,39.63351813324,0.));
#81967=CARTESIAN_POINT('Ctrl Pts',(167.630367150783,40.0156990083359,0.));
#81968=CARTESIAN_POINT('Ctrl Pts',(167.630367150783,40.0156990083359,40.0156990083359));
#81969=CARTESIAN_POINT('Ctrl Pts',(167.630367150783,0.,40.0156990083359));
#81970=CARTESIAN_POINT('Ctrl Pts',(167.630367150783,-40.0156990083359,40.0156990083359));
#81971=CARTESIAN_POINT('Ctrl Pts',(167.630367150783,-40.0156990083359,0.));
#81972=CARTESIAN_POINT('Ctrl Pts',(167.630367150783,-40.0156990083359,-40.0156990083359));
#81973=CARTESIAN_POINT('Ctrl Pts',(167.630367150783,0.,-40.0156990083359));
#81974=CARTESIAN_POINT('Ctrl Pts',(167.630367150783,40.0156990083359,-40.0156990083359));
#81975=CARTESIAN_POINT('Ctrl Pts',(167.630367150783,40.0156990083359,0.));
#81976=CARTESIAN_POINT('Ctrl Pts',(166.993062838849,40.3750959589866,0.));
#81977=CARTESIAN_POINT('Ctrl Pts',(166.993062838849,40.3750959589866,40.3750959589866));
#81978=CARTESIAN_POINT('Ctrl Pts',(166.993062838849,0.,40.3750959589866));
#81979=CARTESIAN_POINT('Ctrl Pts',(166.993062838849,-40.3750959589866,40.3750959589866));
#81980=CARTESIAN_POINT('Ctrl Pts',(166.993062838849,-40.3750959589866,0.));
#81981=CARTESIAN_POINT('Ctrl Pts',(166.993062838849,-40.3750959589866,-40.3750959589866));
#81982=CARTESIAN_POINT('Ctrl Pts',(166.993062838849,0.,-40.3750959589866));
#81983=CARTESIAN_POINT('Ctrl Pts',(166.993062838849,40.3750959589866,-40.3750959589866));
#81984=CARTESIAN_POINT('Ctrl Pts',(166.993062838849,40.3750959589866,0.));
#81985=CARTESIAN_POINT('Ctrl Pts',(166.501725227547,40.6755375400619,0.));
#81986=CARTESIAN_POINT('Ctrl Pts',(166.501725227547,40.6755375400618,40.6755375400618));
#81987=CARTESIAN_POINT('Ctrl Pts',(166.501725227547,0.,40.6755375400619));
#81988=CARTESIAN_POINT('Ctrl Pts',(166.501725227547,-40.6755375400618,40.6755375400618));
#81989=CARTESIAN_POINT('Ctrl Pts',(166.501725227547,-40.6755375400619,0.));
#81990=CARTESIAN_POINT('Ctrl Pts',(166.501725227547,-40.6755375400618,-40.6755375400618));
#81991=CARTESIAN_POINT('Ctrl Pts',(166.501725227547,0.,-40.6755375400619));
#81992=CARTESIAN_POINT('Ctrl Pts',(166.501725227547,40.6755375400618,-40.6755375400618));
#81993=CARTESIAN_POINT('Ctrl Pts',(166.501725227547,40.6755375400619,0.));
#81994=CARTESIAN_POINT('Ctrl Pts',(166.168231046464,40.889558113312,0.));
#81995=CARTESIAN_POINT('Ctrl Pts',(166.168231046464,40.889558113312,40.889558113312));
#81996=CARTESIAN_POINT('Ctrl Pts',(166.168231046464,0.,40.889558113312));
#81997=CARTESIAN_POINT('Ctrl Pts',(166.168231046464,-40.889558113312,40.889558113312));
#81998=CARTESIAN_POINT('Ctrl Pts',(166.168231046464,-40.889558113312,0.));
#81999=CARTESIAN_POINT('Ctrl Pts',(166.168231046464,-40.889558113312,-40.889558113312));
#82000=CARTESIAN_POINT('Ctrl Pts',(166.168231046464,0.,-40.889558113312));
#82001=CARTESIAN_POINT('Ctrl Pts',(166.168231046464,40.889558113312,-40.889558113312));
#82002=CARTESIAN_POINT('Ctrl Pts',(166.168231046464,40.889558113312,0.));
#82003=CARTESIAN_POINT('Ctrl Pts',(166.,41.,0.));
#82004=CARTESIAN_POINT('Ctrl Pts',(166.,41.,41.));
#82005=CARTESIAN_POINT('Ctrl Pts',(166.,0.,41.));
#82006=CARTESIAN_POINT('Ctrl Pts',(166.,-41.,41.));
#82007=CARTESIAN_POINT('Ctrl Pts',(166.,-41.,0.));
#82008=CARTESIAN_POINT('Ctrl Pts',(166.,-41.,-41.));
#82009=CARTESIAN_POINT('Ctrl Pts',(166.,0.,-41.));
#82010=CARTESIAN_POINT('Ctrl Pts',(166.,41.,-41.));
#82011=CARTESIAN_POINT('Ctrl Pts',(166.,41.,0.));
#82012=CARTESIAN_POINT('',(216.,16.5,0.));
#82013=CARTESIAN_POINT('Ctrl Pts',(166.,41.,0.));
#82014=CARTESIAN_POINT('Ctrl Pts',(166.168231046464,40.889558113312,0.));
#82015=CARTESIAN_POINT('Ctrl Pts',(166.501725227547,40.6755375400619,0.));
#82016=CARTESIAN_POINT('Ctrl Pts',(166.993062838849,40.3750959589866,0.));
#82017=CARTESIAN_POINT('Ctrl Pts',(167.630367150783,40.0156990083359,0.));
#82018=CARTESIAN_POINT('Ctrl Pts',(168.397662779334,39.63351813324,0.));
#82019=CARTESIAN_POINT('Ctrl Pts',(169.136715408109,39.3135851151319,0.));
#82020=CARTESIAN_POINT('Ctrl Pts',(169.849764887444,39.0460911245127,0.));
#82021=CARTESIAN_POINT('Ctrl Pts',(170.540530769115,38.8148056986339,0.));
#82022=CARTESIAN_POINT('Ctrl Pts',(171.214744140827,38.5947917128636,0.));
#82023=CARTESIAN_POINT('Ctrl Pts',(171.879381987014,38.35560208533,0.));
#82024=CARTESIAN_POINT('Ctrl Pts',(172.541509808549,38.0660475925471,0.));
#82025=CARTESIAN_POINT('Ctrl Pts',(173.207330843265,37.6982699366733,0.));
#82026=CARTESIAN_POINT('Ctrl Pts',(173.88097676403,37.2324839644745,0.));
#82027=CARTESIAN_POINT('Ctrl Pts',(174.563968613803,36.6602217315156,0.));
#82028=CARTESIAN_POINT('Ctrl Pts',(175.256166976199,35.9845194006668,0.));
#82029=CARTESIAN_POINT('Ctrl Pts',(175.956404761947,35.220592169579,0.));
#82030=CARTESIAN_POINT('Ctrl Pts',(176.663284323105,34.3965983321123,0.));
#82031=CARTESIAN_POINT('Ctrl Pts',(177.375813082222,33.5537582813009,0.));
#82032=CARTESIAN_POINT('Ctrl Pts',(178.094333722328,32.7483045448037,0.));
#82033=CARTESIAN_POINT('Ctrl Pts',(178.82040630265,32.0463508095147,0.));
#82034=CARTESIAN_POINT('Ctrl Pts',(179.555779619084,31.5125164881584,0.));
#82035=CARTESIAN_POINT('Ctrl Pts',(180.301606849543,31.2002008326786,0.));
#82036=CARTESIAN_POINT('Ctrl Pts',(181.057582682021,31.141384874781,0.));
#82037=CARTESIAN_POINT('Ctrl Pts',(181.821060794834,31.336111008946,0.));
#82038=CARTESIAN_POINT('Ctrl Pts',(182.586327425199,31.7435152517629,0.));
#82039=CARTESIAN_POINT('Ctrl Pts',(183.346276790563,32.2953778251868,0.));
#82040=CARTESIAN_POINT('Ctrl Pts',(184.093886879022,32.9080070117905,0.));
#82041=CARTESIAN_POINT('Ctrl Pts',(184.823852750706,33.4950850843424,0.));
#82042=CARTESIAN_POINT('Ctrl Pts',(185.533966240925,33.9792969407959,0.));
#82043=CARTESIAN_POINT('Ctrl Pts',(186.227093638197,34.3065527505812,0.));
#82044=CARTESIAN_POINT('Ctrl Pts',(186.909683874378,34.4456555286542,0.));
#82045=CARTESIAN_POINT('Ctrl Pts',(187.589050043455,34.3832180811066,0.));
#82046=CARTESIAN_POINT('Ctrl Pts',(188.271268152939,34.1203973311724,0.));
#82047=CARTESIAN_POINT('Ctrl Pts',(188.958330678398,33.6683706359231,0.));
#82048=CARTESIAN_POINT('Ctrl Pts',(189.647329687564,33.0461922340397,0.));
#82049=CARTESIAN_POINT('Ctrl Pts',(190.332663752398,32.2818828529496,0.));
#82050=CARTESIAN_POINT('Ctrl Pts',(191.007499403008,31.4126397968556,0.));
#82051=CARTESIAN_POINT('Ctrl Pts',(191.665604121366,30.4857275954352,0.));
#82052=CARTESIAN_POINT('Ctrl Pts',(192.302852321524,29.5583582075276,0.));
#82053=CARTESIAN_POINT('Ctrl Pts',(192.919287538658,28.6998106357671,0.));
#82054=CARTESIAN_POINT('Ctrl Pts',(193.519372459537,27.9858382864175,0.));
#82055=CARTESIAN_POINT('Ctrl Pts',(194.110246528525,27.4849758320246,0.));
#82056=CARTESIAN_POINT('Ctrl Pts',(194.700480719299,27.246160623384,0.));
#82057=CARTESIAN_POINT('Ctrl Pts',(195.298687821752,27.2875376857686,0.));
#82058=CARTESIAN_POINT('Ctrl Pts',(195.912058185941,27.5804806183496,0.));
#82059=CARTESIAN_POINT('Ctrl Pts',(196.545471802854,28.0523886024101,0.));
#82060=CARTESIAN_POINT('Ctrl Pts',(197.201256210244,28.6080668697552,0.));
#82061=CARTESIAN_POINT('Ctrl Pts',(197.878737400882,29.146450351934,0.));
#82062=CARTESIAN_POINT('Ctrl Pts',(198.57393042139,29.5782809062286,0.));
#82063=CARTESIAN_POINT('Ctrl Pts',(199.279015532529,29.8458345487875,0.));
#82064=CARTESIAN_POINT('Ctrl Pts',(199.983241107359,29.9194471715901,0.));
#82065=CARTESIAN_POINT('Ctrl Pts',(200.674069577301,29.7890397540896,0.));
#82066=CARTESIAN_POINT('Ctrl Pts',(201.338274525702,29.4580312858847,0.));
#82067=CARTESIAN_POINT('Ctrl Pts',(201.962968334053,28.934797520153,0.));
#82068=CARTESIAN_POINT('Ctrl Pts',(202.537022078747,28.231020604859,0.));
#82069=CARTESIAN_POINT('Ctrl Pts',(203.052959516359,27.3665743841578,0.));
#82070=CARTESIAN_POINT('Ctrl Pts',(203.508634483801,26.3724343604023,0.));
#82071=CARTESIAN_POINT('Ctrl Pts',(203.909197365198,25.2948962814451,0.));
#82072=CARTESIAN_POINT('Ctrl Pts',(204.268492247486,24.1981104944312,0.));
#82073=CARTESIAN_POINT('Ctrl Pts',(204.611869907935,23.1702821776947,0.));
#82074=CARTESIAN_POINT('Ctrl Pts',(204.97132698008,22.3105170035492,0.));
#82075=CARTESIAN_POINT('Ctrl Pts',(205.378164090918,21.7094404040115,0.));
#82076=CARTESIAN_POINT('Ctrl Pts',(205.856117010386,21.4309931834381,0.));
#82077=CARTESIAN_POINT('Ctrl Pts',(206.415057633172,21.495656810279,0.));
#82078=CARTESIAN_POINT('Ctrl Pts',(207.042444432711,21.858011778557,0.));
#82079=CARTESIAN_POINT('Ctrl Pts',(207.709418184682,22.4211128317459,0.));
#82080=CARTESIAN_POINT('Ctrl Pts',(208.381214512496,23.0617114361388,0.));
#82081=CARTESIAN_POINT('Ctrl Pts',(209.02608343001,23.651711850736,0.));
#82082=CARTESIAN_POINT('Ctrl Pts',(209.624909485776,24.0813843942427,0.));
#82083=CARTESIAN_POINT('Ctrl Pts',(210.180310680863,24.2813063241724,0.));
#82084=CARTESIAN_POINT('Ctrl Pts',(210.707332937096,24.2178287727218,0.));
#82085=CARTESIAN_POINT('Ctrl Pts',(211.225193342687,23.8887926005784,0.));
#82086=CARTESIAN_POINT('Ctrl Pts',(211.747183985356,23.3196384840519,0.));
#82087=CARTESIAN_POINT('Ctrl Pts',(212.2765623513,22.557779972217,0.));
#82088=CARTESIAN_POINT('Ctrl Pts',(212.810267068812,21.6644655526099,0.));
#82089=CARTESIAN_POINT('Ctrl Pts',(213.340647821643,20.70741247154,0.));
#82090=CARTESIAN_POINT('Ctrl Pts',(213.858063274574,19.7528683772512,0.));
#82091=CARTESIAN_POINT('Ctrl Pts',(214.352945230993,18.8585426236962,0.));
#82092=CARTESIAN_POINT('Ctrl Pts',(214.818499221249,18.0645628079122,0.));
#82093=CARTESIAN_POINT('Ctrl Pts',(215.250787804816,17.3944424189593,0.));
#82094=CARTESIAN_POINT('Ctrl Pts',(215.568414172701,16.9669101302242,0.));
#82095=CARTESIAN_POINT('Ctrl Pts',(215.790485987678,16.7090430293136,0.));
#82096=CARTESIAN_POINT('Ctrl Pts',(215.931357948425,16.5650312142703,0.));
#82097=CARTESIAN_POINT('Ctrl Pts',(216.,16.5,0.));
#82098=CARTESIAN_POINT('',(216.,-16.5,-2.02066721859313E-15));
#82099=CARTESIAN_POINT('Origin',(216.,0.,0.));
#82100=CARTESIAN_POINT('Origin',(216.,0.,0.));
#82101=CARTESIAN_POINT('Origin',(216.5,0.,0.));
#82102=CARTESIAN_POINT('',(217.,-14.,-1.71450551880629E-15));
#82103=CARTESIAN_POINT('Origin',(217.,0.,0.));
#82104=CARTESIAN_POINT('',(216.5,-15.25,-1.86758636869971E-15));
#82105=CARTESIAN_POINT('Origin',(223.5,0.,0.));
#82106=CARTESIAN_POINT('',(230.,-14.,-1.71450551880629E-15));
#82107=CARTESIAN_POINT('Origin',(230.,0.,0.));
#82108=CARTESIAN_POINT('',(223.5,-14.,-1.71450551880629E-15));
#82109=CARTESIAN_POINT('Origin',(230.,12.,0.));
#82110=CARTESIAN_POINT('',(230.,-12.,-1.46957615897682E-15));
#82111=CARTESIAN_POINT('Origin',(230.,0.,0.));
#82112=CARTESIAN_POINT('Origin',(223.,0.,0.));
#82113=CARTESIAN_POINT('',(216.,-12.,-1.46957615897682E-15));
#82114=CARTESIAN_POINT('',(223.,-12.,-1.46957615897682E-15));
#82115=CARTESIAN_POINT('Origin',(216.,0.,0.));
#82116=CARTESIAN_POINT('Origin',(216.,14.,0.));
#82117=CARTESIAN_POINT('',(216.,14.,0.));
#82118=CARTESIAN_POINT('Origin',(216.,0.,0.));
#82119=CARTESIAN_POINT('Ctrl Pts',(166.5,38.5,0.));
#82120=CARTESIAN_POINT('Ctrl Pts',(166.5,38.5,38.5));
#82121=CARTESIAN_POINT('Ctrl Pts',(166.5,0.,38.5));
#82122=CARTESIAN_POINT('Ctrl Pts',(166.5,-38.5,38.5));
#82123=CARTESIAN_POINT('Ctrl Pts',(166.5,-38.5,0.));
#82124=CARTESIAN_POINT('Ctrl Pts',(166.5,-38.5,-38.5));
#82125=CARTESIAN_POINT('Ctrl Pts',(166.5,0.,-38.5));
#82126=CARTESIAN_POINT('Ctrl Pts',(166.5,38.5,-38.5));
#82127=CARTESIAN_POINT('Ctrl Pts',(166.5,38.5,0.));
#82128=CARTESIAN_POINT('Ctrl Pts',(166.646027830324,38.384297265584,0.));
#82129=CARTESIAN_POINT('Ctrl Pts',(166.646027830324,38.384297265584,38.384297265584));
#82130=CARTESIAN_POINT('Ctrl Pts',(166.646027830324,0.,38.384297265584));
#82131=CARTESIAN_POINT('Ctrl Pts',(166.646027830324,-38.384297265584,38.384297265584));
#82132=CARTESIAN_POINT('Ctrl Pts',(166.646027830324,-38.384297265584,0.));
#82133=CARTESIAN_POINT('Ctrl Pts',(166.646027830324,-38.384297265584,-38.384297265584));
#82134=CARTESIAN_POINT('Ctrl Pts',(166.646027830324,0.,-38.384297265584));
#82135=CARTESIAN_POINT('Ctrl Pts',(166.646027830324,38.384297265584,-38.384297265584));
#82136=CARTESIAN_POINT('Ctrl Pts',(166.646027830324,38.384297265584,0.));
#82137=CARTESIAN_POINT('Ctrl Pts',(166.936935989037,38.1603786909402,0.));
#82138=CARTESIAN_POINT('Ctrl Pts',(166.936935989037,38.1603786909402,38.1603786909402));
#82139=CARTESIAN_POINT('Ctrl Pts',(166.936935989037,0.,38.1603786909402));
#82140=CARTESIAN_POINT('Ctrl Pts',(166.936935989037,-38.1603786909402,38.1603786909402));
#82141=CARTESIAN_POINT('Ctrl Pts',(166.936935989037,-38.1603786909402,0.));
#82142=CARTESIAN_POINT('Ctrl Pts',(166.936935989037,-38.1603786909402,-38.1603786909402));
#82143=CARTESIAN_POINT('Ctrl Pts',(166.936935989037,0.,-38.1603786909402));
#82144=CARTESIAN_POINT('Ctrl Pts',(166.936935989037,38.1603786909402,-38.1603786909402));
#82145=CARTESIAN_POINT('Ctrl Pts',(166.936935989037,38.1603786909402,0.));
#82146=CARTESIAN_POINT('Ctrl Pts',(167.369855715636,37.8469615594215,0.));
#82147=CARTESIAN_POINT('Ctrl Pts',(167.369855715636,37.8469615594215,37.8469615594215));
#82148=CARTESIAN_POINT('Ctrl Pts',(167.369855715636,0.,37.8469615594215));
#82149=CARTESIAN_POINT('Ctrl Pts',(167.369855715636,-37.8469615594215,37.8469615594215));
#82150=CARTESIAN_POINT('Ctrl Pts',(167.369855715636,-37.8469615594215,0.));
#82151=CARTESIAN_POINT('Ctrl Pts',(167.369855715636,-37.8469615594215,-37.8469615594215));
#82152=CARTESIAN_POINT('Ctrl Pts',(167.369855715636,0.,-37.8469615594215));
#82153=CARTESIAN_POINT('Ctrl Pts',(167.369855715636,37.8469615594215,-37.8469615594215));
#82154=CARTESIAN_POINT('Ctrl Pts',(167.369855715636,37.8469615594215,0.));
#82155=CARTESIAN_POINT('Ctrl Pts',(167.940195292269,37.4740045272214,0.));
#82156=CARTESIAN_POINT('Ctrl Pts',(167.940195292269,37.4740045272214,37.4740045272214));
#82157=CARTESIAN_POINT('Ctrl Pts',(167.940195292269,0.,37.4740045272214));
#82158=CARTESIAN_POINT('Ctrl Pts',(167.940195292269,-37.4740045272214,37.4740045272214));
#82159=CARTESIAN_POINT('Ctrl Pts',(167.940195292269,-37.4740045272214,0.));
#82160=CARTESIAN_POINT('Ctrl Pts',(167.940195292269,-37.4740045272214,-37.4740045272214));
#82161=CARTESIAN_POINT('Ctrl Pts',(167.940195292269,0.,-37.4740045272214));
#82162=CARTESIAN_POINT('Ctrl Pts',(167.940195292269,37.4740045272214,-37.4740045272214));
#82163=CARTESIAN_POINT('Ctrl Pts',(167.940195292269,37.4740045272214,0.));
#82164=CARTESIAN_POINT('Ctrl Pts',(168.641815524474,37.0808938108885,0.));
#82165=CARTESIAN_POINT('Ctrl Pts',(168.641815524474,37.0808938108885,37.0808938108885));
#82166=CARTESIAN_POINT('Ctrl Pts',(168.641815524474,0.,37.0808938108885));
#82167=CARTESIAN_POINT('Ctrl Pts',(168.641815524474,-37.0808938108885,37.0808938108885));
#82168=CARTESIAN_POINT('Ctrl Pts',(168.641815524474,-37.0808938108885,0.));
#82169=CARTESIAN_POINT('Ctrl Pts',(168.641815524474,-37.0808938108885,-37.0808938108885));
#82170=CARTESIAN_POINT('Ctrl Pts',(168.641815524474,0.,-37.0808938108885));
#82171=CARTESIAN_POINT('Ctrl Pts',(168.641815524474,37.0808938108885,-37.0808938108885));
#82172=CARTESIAN_POINT('Ctrl Pts',(168.641815524474,37.0808938108885,0.));
#82173=CARTESIAN_POINT('Ctrl Pts',(169.332671034328,36.7553393532152,0.));
#82174=CARTESIAN_POINT('Ctrl Pts',(169.332671034328,36.7553393532152,36.7553393532152));
#82175=CARTESIAN_POINT('Ctrl Pts',(169.332671034328,0.,36.7553393532152));
#82176=CARTESIAN_POINT('Ctrl Pts',(169.332671034328,-36.7553393532152,36.7553393532152));
#82177=CARTESIAN_POINT('Ctrl Pts',(169.332671034328,-36.7553393532152,0.));
#82178=CARTESIAN_POINT('Ctrl Pts',(169.332671034328,-36.7553393532152,-36.7553393532152));
#82179=CARTESIAN_POINT('Ctrl Pts',(169.332671034328,0.,-36.7553393532152));
#82180=CARTESIAN_POINT('Ctrl Pts',(169.332671034328,36.7553393532152,-36.7553393532152));
#82181=CARTESIAN_POINT('Ctrl Pts',(169.332671034328,36.7553393532152,0.));
#82182=CARTESIAN_POINT('Ctrl Pts',(170.013852859503,36.4862057554389,0.));
#82183=CARTESIAN_POINT('Ctrl Pts',(170.013852859503,36.4862057554389,36.4862057554389));
#82184=CARTESIAN_POINT('Ctrl Pts',(170.013852859503,0.,36.4862057554389));
#82185=CARTESIAN_POINT('Ctrl Pts',(170.013852859503,-36.4862057554389,36.4862057554389));
#82186=CARTESIAN_POINT('Ctrl Pts',(170.013852859503,-36.4862057554389,0.));
#82187=CARTESIAN_POINT('Ctrl Pts',(170.013852859503,-36.4862057554389,-36.4862057554389));
#82188=CARTESIAN_POINT('Ctrl Pts',(170.013852859503,0.,-36.4862057554389));
#82189=CARTESIAN_POINT('Ctrl Pts',(170.013852859503,36.4862057554389,-36.4862057554389));
#82190=CARTESIAN_POINT('Ctrl Pts',(170.013852859503,36.4862057554389,0.));
#82191=CARTESIAN_POINT('Ctrl Pts',(170.687195598755,36.25481814225,0.));
#82192=CARTESIAN_POINT('Ctrl Pts',(170.687195598755,36.25481814225,36.25481814225));
#82193=CARTESIAN_POINT('Ctrl Pts',(170.687195598755,0.,36.25481814225));
#82194=CARTESIAN_POINT('Ctrl Pts',(170.687195598755,-36.25481814225,36.25481814225));
#82195=CARTESIAN_POINT('Ctrl Pts',(170.687195598755,-36.25481814225,0.));
#82196=CARTESIAN_POINT('Ctrl Pts',(170.687195598755,-36.25481814225,-36.25481814225));
#82197=CARTESIAN_POINT('Ctrl Pts',(170.687195598755,0.,-36.25481814225));
#82198=CARTESIAN_POINT('Ctrl Pts',(170.687195598755,36.25481814225,-36.25481814225));
#82199=CARTESIAN_POINT('Ctrl Pts',(170.687195598755,36.25481814225,0.));
#82200=CARTESIAN_POINT('Ctrl Pts',(171.355454837575,36.0331538549227,0.));
#82201=CARTESIAN_POINT('Ctrl Pts',(171.355454837575,36.0331538549227,36.0331538549227));
#82202=CARTESIAN_POINT('Ctrl Pts',(171.355454837575,0.,36.0331538549227));
#82203=CARTESIAN_POINT('Ctrl Pts',(171.355454837575,-36.0331538549227,36.0331538549227));
#82204=CARTESIAN_POINT('Ctrl Pts',(171.355454837575,-36.0331538549227,0.));
#82205=CARTESIAN_POINT('Ctrl Pts',(171.355454837575,-36.0331538549227,-36.0331538549227));
#82206=CARTESIAN_POINT('Ctrl Pts',(171.355454837575,0.,-36.0331538549227));
#82207=CARTESIAN_POINT('Ctrl Pts',(171.355454837575,36.0331538549227,-36.0331538549227));
#82208=CARTESIAN_POINT('Ctrl Pts',(171.355454837575,36.0331538549227,0.));
#82209=CARTESIAN_POINT('Ctrl Pts',(172.021839116729,35.7885524264098,0.));
#82210=CARTESIAN_POINT('Ctrl Pts',(172.021839116729,35.7885524264098,35.7885524264098));
#82211=CARTESIAN_POINT('Ctrl Pts',(172.021839116729,0.,35.7885524264098));
#82212=CARTESIAN_POINT('Ctrl Pts',(172.021839116729,-35.7885524264098,35.7885524264098));
#82213=CARTESIAN_POINT('Ctrl Pts',(172.021839116729,-35.7885524264098,0.));
#82214=CARTESIAN_POINT('Ctrl Pts',(172.021839116729,-35.7885524264098,-35.7885524264098));
#82215=CARTESIAN_POINT('Ctrl Pts',(172.021839116729,0.,-35.7885524264098));
#82216=CARTESIAN_POINT('Ctrl Pts',(172.021839116729,35.7885524264098,-35.7885524264098));
#82217=CARTESIAN_POINT('Ctrl Pts',(172.021839116729,35.7885524264098,0.));
#82218=CARTESIAN_POINT('Ctrl Pts',(172.689527753591,35.4884519662692,0.));
#82219=CARTESIAN_POINT('Ctrl Pts',(172.689527753591,35.4884519662692,35.4884519662692));
#82220=CARTESIAN_POINT('Ctrl Pts',(172.689527753591,0.,35.4884519662692));
#82221=CARTESIAN_POINT('Ctrl Pts',(172.689527753591,-35.4884519662692,35.4884519662692));
#82222=CARTESIAN_POINT('Ctrl Pts',(172.689527753591,-35.4884519662692,0.));
#82223=CARTESIAN_POINT('Ctrl Pts',(172.689527753591,-35.4884519662692,-35.4884519662692));
#82224=CARTESIAN_POINT('Ctrl Pts',(172.689527753591,0.,-35.4884519662692));
#82225=CARTESIAN_POINT('Ctrl Pts',(172.689527753591,35.4884519662692,-35.4884519662692));
#82226=CARTESIAN_POINT('Ctrl Pts',(172.689527753591,35.4884519662692,0.));
#82227=CARTESIAN_POINT('Ctrl Pts',(173.361242516346,35.1048554959833,0.));
#82228=CARTESIAN_POINT('Ctrl Pts',(173.361242516346,35.1048554959833,35.1048554959833));
#82229=CARTESIAN_POINT('Ctrl Pts',(173.361242516346,0.,35.1048554959833));
#82230=CARTESIAN_POINT('Ctrl Pts',(173.361242516346,-35.1048554959833,35.1048554959833));
#82231=CARTESIAN_POINT('Ctrl Pts',(173.361242516346,-35.1048554959833,0.));
#82232=CARTESIAN_POINT('Ctrl Pts',(173.361242516346,-35.1048554959833,-35.1048554959833));
#82233=CARTESIAN_POINT('Ctrl Pts',(173.361242516346,0.,-35.1048554959833));
#82234=CARTESIAN_POINT('Ctrl Pts',(173.361242516346,35.1048554959833,-35.1048554959833));
#82235=CARTESIAN_POINT('Ctrl Pts',(173.361242516346,35.1048554959833,0.));
#82236=CARTESIAN_POINT('Ctrl Pts',(174.038678741555,34.6195419357237,0.));
#82237=CARTESIAN_POINT('Ctrl Pts',(174.038678741555,34.6195419357237,34.6195419357237));
#82238=CARTESIAN_POINT('Ctrl Pts',(174.038678741555,0.,34.6195419357237));
#82239=CARTESIAN_POINT('Ctrl Pts',(174.038678741555,-34.6195419357237,34.6195419357237));
#82240=CARTESIAN_POINT('Ctrl Pts',(174.038678741555,-34.6195419357237,0.));
#82241=CARTESIAN_POINT('Ctrl Pts',(174.038678741555,-34.6195419357237,-34.6195419357237));
#82242=CARTESIAN_POINT('Ctrl Pts',(174.038678741555,0.,-34.6195419357237));
#82243=CARTESIAN_POINT('Ctrl Pts',(174.038678741555,34.6195419357237,-34.6195419357237));
#82244=CARTESIAN_POINT('Ctrl Pts',(174.038678741555,34.6195419357237,0.));
#82245=CARTESIAN_POINT('Ctrl Pts',(174.722485008373,34.0263777716625,0.));
#82246=CARTESIAN_POINT('Ctrl Pts',(174.722485008373,34.0263777716625,34.0263777716625));
#82247=CARTESIAN_POINT('Ctrl Pts',(174.722485008373,0.,34.0263777716625));
#82248=CARTESIAN_POINT('Ctrl Pts',(174.722485008373,-34.0263777716625,34.0263777716625));
#82249=CARTESIAN_POINT('Ctrl Pts',(174.722485008373,-34.0263777716625,0.));
#82250=CARTESIAN_POINT('Ctrl Pts',(174.722485008373,-34.0263777716625,-34.0263777716625));
#82251=CARTESIAN_POINT('Ctrl Pts',(174.722485008373,0.,-34.0263777716625));
#82252=CARTESIAN_POINT('Ctrl Pts',(174.722485008373,34.0263777716625,-34.0263777716625));
#82253=CARTESIAN_POINT('Ctrl Pts',(174.722485008373,34.0263777716625,0.));
#82254=CARTESIAN_POINT('Ctrl Pts',(175.412716697241,33.3312296578559,0.));
#82255=CARTESIAN_POINT('Ctrl Pts',(175.412716697241,33.3312296578559,33.3312296578559));
#82256=CARTESIAN_POINT('Ctrl Pts',(175.412716697241,0.,33.3312296578559));
#82257=CARTESIAN_POINT('Ctrl Pts',(175.412716697241,-33.3312296578559,33.3312296578559));
#82258=CARTESIAN_POINT('Ctrl Pts',(175.412716697241,-33.3312296578559,0.));
#82259=CARTESIAN_POINT('Ctrl Pts',(175.412716697241,-33.3312296578559,-33.3312296578559));
#82260=CARTESIAN_POINT('Ctrl Pts',(175.412716697241,0.,-33.3312296578559));
#82261=CARTESIAN_POINT('Ctrl Pts',(175.412716697241,33.3312296578559,-33.3312296578559));
#82262=CARTESIAN_POINT('Ctrl Pts',(175.412716697241,33.3312296578559,0.));
#82263=CARTESIAN_POINT('Ctrl Pts',(176.10914445329,32.5524621154421,0.));
#82264=CARTESIAN_POINT('Ctrl Pts',(176.10914445329,32.5524621154421,32.5524621154421));
#82265=CARTESIAN_POINT('Ctrl Pts',(176.10914445329,0.,32.5524621154421));
#82266=CARTESIAN_POINT('Ctrl Pts',(176.10914445329,-32.5524621154421,32.5524621154421));
#82267=CARTESIAN_POINT('Ctrl Pts',(176.10914445329,-32.5524621154421,0.));
#82268=CARTESIAN_POINT('Ctrl Pts',(176.10914445329,-32.5524621154421,-32.5524621154421));
#82269=CARTESIAN_POINT('Ctrl Pts',(176.10914445329,0.,-32.5524621154421));
#82270=CARTESIAN_POINT('Ctrl Pts',(176.10914445329,32.5524621154421,-32.5524621154421));
#82271=CARTESIAN_POINT('Ctrl Pts',(176.10914445329,32.5524621154421,0.));
#82272=CARTESIAN_POINT('Ctrl Pts',(176.811644553588,31.7214384106704,0.));
#82273=CARTESIAN_POINT('Ctrl Pts',(176.811644553588,31.7214384106704,31.7214384106704));
#82274=CARTESIAN_POINT('Ctrl Pts',(176.811644553588,0.,31.7214384106704));
#82275=CARTESIAN_POINT('Ctrl Pts',(176.811644553588,-31.7214384106704,31.7214384106704));
#82276=CARTESIAN_POINT('Ctrl Pts',(176.811644553588,-31.7214384106704,0.));
#82277=CARTESIAN_POINT('Ctrl Pts',(176.811644553588,-31.7214384106704,-31.7214384106704));
#82278=CARTESIAN_POINT('Ctrl Pts',(176.811644553588,0.,-31.7214384106704));
#82279=CARTESIAN_POINT('Ctrl Pts',(176.811644553588,31.7214384106704,-31.7214384106704));
#82280=CARTESIAN_POINT('Ctrl Pts',(176.811644553588,31.7214384106704,0.));
#82281=CARTESIAN_POINT('Ctrl Pts',(177.520501166053,30.8825005559741,0.));
#82282=CARTESIAN_POINT('Ctrl Pts',(177.520501166053,30.882500555974,30.882500555974));
#82283=CARTESIAN_POINT('Ctrl Pts',(177.520501166053,0.,30.8825005559741));
#82284=CARTESIAN_POINT('Ctrl Pts',(177.520501166053,-30.882500555974,30.882500555974));
#82285=CARTESIAN_POINT('Ctrl Pts',(177.520501166053,-30.8825005559741,0.));
#82286=CARTESIAN_POINT('Ctrl Pts',(177.520501166053,-30.882500555974,-30.882500555974));
#82287=CARTESIAN_POINT('Ctrl Pts',(177.520501166053,0.,-30.8825005559741));
#82288=CARTESIAN_POINT('Ctrl Pts',(177.520501166053,30.882500555974,-30.882500555974));
#82289=CARTESIAN_POINT('Ctrl Pts',(177.520501166053,30.8825005559741,0.));
#82290=CARTESIAN_POINT('Ctrl Pts',(178.236882848697,30.0945584620795,0.));
#82291=CARTESIAN_POINT('Ctrl Pts',(178.236882848697,30.0945584620794,30.0945584620794));
#82292=CARTESIAN_POINT('Ctrl Pts',(178.236882848697,0.,30.0945584620795));
#82293=CARTESIAN_POINT('Ctrl Pts',(178.236882848697,-30.0945584620794,30.0945584620794));
#82294=CARTESIAN_POINT('Ctrl Pts',(178.236882848697,-30.0945584620795,0.));
#82295=CARTESIAN_POINT('Ctrl Pts',(178.236882848697,-30.0945584620794,-30.0945584620794));
#82296=CARTESIAN_POINT('Ctrl Pts',(178.236882848697,0.,-30.0945584620795));
#82297=CARTESIAN_POINT('Ctrl Pts',(178.236882848697,30.0945584620794,-30.0945584620794));
#82298=CARTESIAN_POINT('Ctrl Pts',(178.236882848697,30.0945584620795,0.));
#82299=CARTESIAN_POINT('Ctrl Pts',(178.962404276569,29.4235353639997,0.));
#82300=CARTESIAN_POINT('Ctrl Pts',(178.962404276569,29.4235353639996,29.4235353639996));
#82301=CARTESIAN_POINT('Ctrl Pts',(178.962404276569,0.,29.4235353639997));
#82302=CARTESIAN_POINT('Ctrl Pts',(178.962404276569,-29.4235353639996,29.4235353639996));
#82303=CARTESIAN_POINT('Ctrl Pts',(178.962404276569,-29.4235353639997,0.));
#82304=CARTESIAN_POINT('Ctrl Pts',(178.962404276569,-29.4235353639996,-29.4235353639996));
#82305=CARTESIAN_POINT('Ctrl Pts',(178.962404276569,0.,-29.4235353639997));
#82306=CARTESIAN_POINT('Ctrl Pts',(178.962404276569,29.4235353639996,-29.4235353639996));
#82307=CARTESIAN_POINT('Ctrl Pts',(178.962404276569,29.4235353639997,0.));
#82308=CARTESIAN_POINT('Ctrl Pts',(179.69839696542,28.9318633546098,0.));
#82309=CARTESIAN_POINT('Ctrl Pts',(179.69839696542,28.9318633546098,28.9318633546098));
#82310=CARTESIAN_POINT('Ctrl Pts',(179.69839696542,0.,28.9318633546098));
#82311=CARTESIAN_POINT('Ctrl Pts',(179.69839696542,-28.9318633546098,28.9318633546098));
#82312=CARTESIAN_POINT('Ctrl Pts',(179.69839696542,-28.9318633546098,0.));
#82313=CARTESIAN_POINT('Ctrl Pts',(179.69839696542,-28.9318633546098,-28.9318633546098));
#82314=CARTESIAN_POINT('Ctrl Pts',(179.69839696542,0.,-28.9318633546098));
#82315=CARTESIAN_POINT('Ctrl Pts',(179.69839696542,28.9318633546098,-28.9318633546098));
#82316=CARTESIAN_POINT('Ctrl Pts',(179.69839696542,28.9318633546098,0.));
#82317=CARTESIAN_POINT('Ctrl Pts',(180.445242944925,28.6686083897625,0.));
#82318=CARTESIAN_POINT('Ctrl Pts',(180.445242944925,28.6686083897625,28.6686083897625));
#82319=CARTESIAN_POINT('Ctrl Pts',(180.445242944925,0.,28.6686083897625));
#82320=CARTESIAN_POINT('Ctrl Pts',(180.445242944925,-28.6686083897625,28.6686083897625));
#82321=CARTESIAN_POINT('Ctrl Pts',(180.445242944925,-28.6686083897625,0.));
#82322=CARTESIAN_POINT('Ctrl Pts',(180.445242944925,-28.6686083897625,-28.6686083897625));
#82323=CARTESIAN_POINT('Ctrl Pts',(180.445242944925,0.,-28.6686083897625));
#82324=CARTESIAN_POINT('Ctrl Pts',(180.445242944925,28.6686083897625,-28.6686083897625));
#82325=CARTESIAN_POINT('Ctrl Pts',(180.445242944925,28.6686083897625,0.));
#82326=CARTESIAN_POINT('Ctrl Pts',(181.201754230035,28.660085613321,0.));
#82327=CARTESIAN_POINT('Ctrl Pts',(181.201754230035,28.660085613321,28.660085613321));
#82328=CARTESIAN_POINT('Ctrl Pts',(181.201754230035,0.,28.660085613321));
#82329=CARTESIAN_POINT('Ctrl Pts',(181.201754230035,-28.660085613321,28.660085613321));
#82330=CARTESIAN_POINT('Ctrl Pts',(181.201754230035,-28.660085613321,0.));
#82331=CARTESIAN_POINT('Ctrl Pts',(181.201754230035,-28.660085613321,-28.660085613321));
#82332=CARTESIAN_POINT('Ctrl Pts',(181.201754230035,0.,-28.660085613321));
#82333=CARTESIAN_POINT('Ctrl Pts',(181.201754230035,28.660085613321,-28.660085613321));
#82334=CARTESIAN_POINT('Ctrl Pts',(181.201754230035,28.660085613321,0.));
#82335=CARTESIAN_POINT('Ctrl Pts',(181.964356356054,28.8984085343652,0.));
#82336=CARTESIAN_POINT('Ctrl Pts',(181.964356356054,28.8984085343652,28.8984085343652));
#82337=CARTESIAN_POINT('Ctrl Pts',(181.964356356054,0.,28.8984085343652));
#82338=CARTESIAN_POINT('Ctrl Pts',(181.964356356054,-28.8984085343652,28.8984085343652));
#82339=CARTESIAN_POINT('Ctrl Pts',(181.964356356054,-28.8984085343652,0.));
#82340=CARTESIAN_POINT('Ctrl Pts',(181.964356356054,-28.8984085343652,-28.8984085343652));
#82341=CARTESIAN_POINT('Ctrl Pts',(181.964356356054,0.,-28.8984085343652));
#82342=CARTESIAN_POINT('Ctrl Pts',(181.964356356054,28.8984085343652,-28.8984085343652));
#82343=CARTESIAN_POINT('Ctrl Pts',(181.964356356054,28.8984085343652,0.));
#82344=CARTESIAN_POINT('Ctrl Pts',(182.726909789558,29.3367202018516,0.));
#82345=CARTESIAN_POINT('Ctrl Pts',(182.726909789558,29.3367202018516,29.3367202018516));
#82346=CARTESIAN_POINT('Ctrl Pts',(182.726909789558,0.,29.3367202018516));
#82347=CARTESIAN_POINT('Ctrl Pts',(182.726909789558,-29.3367202018516,29.3367202018516));
#82348=CARTESIAN_POINT('Ctrl Pts',(182.726909789558,-29.3367202018516,0.));
#82349=CARTESIAN_POINT('Ctrl Pts',(182.726909789558,-29.3367202018516,-29.3367202018516));
#82350=CARTESIAN_POINT('Ctrl Pts',(182.726909789558,0.,-29.3367202018516));
#82351=CARTESIAN_POINT('Ctrl Pts',(182.726909789558,29.3367202018516,-29.3367202018516));
#82352=CARTESIAN_POINT('Ctrl Pts',(182.726909789558,29.3367202018516,0.));
#82353=CARTESIAN_POINT('Ctrl Pts',(183.482400836276,29.9039282850736,0.));
#82354=CARTESIAN_POINT('Ctrl Pts',(183.482400836276,29.9039282850735,29.9039282850735));
#82355=CARTESIAN_POINT('Ctrl Pts',(183.482400836276,0.,29.9039282850736));
#82356=CARTESIAN_POINT('Ctrl Pts',(183.482400836276,-29.9039282850735,29.9039282850735));
#82357=CARTESIAN_POINT('Ctrl Pts',(183.482400836276,-29.9039282850736,0.));
#82358=CARTESIAN_POINT('Ctrl Pts',(183.482400836276,-29.9039282850735,-29.9039282850735));
#82359=CARTESIAN_POINT('Ctrl Pts',(183.482400836276,0.,-29.9039282850736));
#82360=CARTESIAN_POINT('Ctrl Pts',(183.482400836276,29.9039282850735,-29.9039282850735));
#82361=CARTESIAN_POINT('Ctrl Pts',(183.482400836276,29.9039282850736,0.));
#82362=CARTESIAN_POINT('Ctrl Pts',(184.224280732459,30.5158363027008,0.));
#82363=CARTESIAN_POINT('Ctrl Pts',(184.224280732459,30.5158363027008,30.5158363027008));
#82364=CARTESIAN_POINT('Ctrl Pts',(184.224280732459,0.,30.5158363027008));
#82365=CARTESIAN_POINT('Ctrl Pts',(184.224280732459,-30.5158363027008,30.5158363027008));
#82366=CARTESIAN_POINT('Ctrl Pts',(184.224280732459,-30.5158363027008,0.));
#82367=CARTESIAN_POINT('Ctrl Pts',(184.224280732459,-30.5158363027008,-30.5158363027008));
#82368=CARTESIAN_POINT('Ctrl Pts',(184.224280732459,0.,-30.5158363027008));
#82369=CARTESIAN_POINT('Ctrl Pts',(184.224280732459,30.5158363027008,-30.5158363027008));
#82370=CARTESIAN_POINT('Ctrl Pts',(184.224280732459,30.5158363027008,0.));
#82371=CARTESIAN_POINT('Ctrl Pts',(184.947972925117,31.0878161213455,0.));
#82372=CARTESIAN_POINT('Ctrl Pts',(184.947972925117,31.0878161213455,31.0878161213455));
#82373=CARTESIAN_POINT('Ctrl Pts',(184.947972925117,0.,31.0878161213455));
#82374=CARTESIAN_POINT('Ctrl Pts',(184.947972925117,-31.0878161213455,31.0878161213455));
#82375=CARTESIAN_POINT('Ctrl Pts',(184.947972925117,-31.0878161213455,0.));
#82376=CARTESIAN_POINT('Ctrl Pts',(184.947972925117,-31.0878161213455,-31.0878161213455));
#82377=CARTESIAN_POINT('Ctrl Pts',(184.947972925117,0.,-31.0878161213455));
#82378=CARTESIAN_POINT('Ctrl Pts',(184.947972925117,31.0878161213455,-31.0878161213455));
#82379=CARTESIAN_POINT('Ctrl Pts',(184.947972925117,31.0878161213455,0.));
#82380=CARTESIAN_POINT('Ctrl Pts',(185.652242796566,31.546505030526,0.));
#82381=CARTESIAN_POINT('Ctrl Pts',(185.652242796566,31.546505030526,31.546505030526));
#82382=CARTESIAN_POINT('Ctrl Pts',(185.652242796566,0.,31.546505030526));
#82383=CARTESIAN_POINT('Ctrl Pts',(185.652242796566,-31.546505030526,31.546505030526));
#82384=CARTESIAN_POINT('Ctrl Pts',(185.652242796566,-31.546505030526,0.));
#82385=CARTESIAN_POINT('Ctrl Pts',(185.652242796566,-31.546505030526,-31.546505030526));
#82386=CARTESIAN_POINT('Ctrl Pts',(185.652242796566,0.,-31.546505030526));
#82387=CARTESIAN_POINT('Ctrl Pts',(185.652242796566,31.546505030526,-31.546505030526));
#82388=CARTESIAN_POINT('Ctrl Pts',(185.652242796566,31.546505030526,0.));
#82389=CARTESIAN_POINT('Ctrl Pts',(186.340814647256,31.8427771137434,0.));
#82390=CARTESIAN_POINT('Ctrl Pts',(186.340814647256,31.8427771137434,31.8427771137434));
#82391=CARTESIAN_POINT('Ctrl Pts',(186.340814647256,0.,31.8427771137434));
#82392=CARTESIAN_POINT('Ctrl Pts',(186.340814647256,-31.8427771137434,31.8427771137434));
#82393=CARTESIAN_POINT('Ctrl Pts',(186.340814647256,-31.8427771137434,0.));
#82394=CARTESIAN_POINT('Ctrl Pts',(186.340814647256,-31.8427771137434,-31.8427771137434));
#82395=CARTESIAN_POINT('Ctrl Pts',(186.340814647256,0.,-31.8427771137434));
#82396=CARTESIAN_POINT('Ctrl Pts',(186.340814647256,31.8427771137434,-31.8427771137434));
#82397=CARTESIAN_POINT('Ctrl Pts',(186.340814647256,31.8427771137434,0.));
#82398=CARTESIAN_POINT('Ctrl Pts',(187.020322757229,31.9488468045685,0.));
#82399=CARTESIAN_POINT('Ctrl Pts',(187.020322757229,31.9488468045685,31.9488468045685));
#82400=CARTESIAN_POINT('Ctrl Pts',(187.020322757229,0.,31.9488468045685));
#82401=CARTESIAN_POINT('Ctrl Pts',(187.020322757229,-31.9488468045685,31.9488468045685));
#82402=CARTESIAN_POINT('Ctrl Pts',(187.020322757229,-31.9488468045685,0.));
#82403=CARTESIAN_POINT('Ctrl Pts',(187.020322757229,-31.9488468045685,-31.9488468045685));
#82404=CARTESIAN_POINT('Ctrl Pts',(187.020322757229,0.,-31.9488468045685));
#82405=CARTESIAN_POINT('Ctrl Pts',(187.020322757229,31.9488468045685,-31.9488468045685));
#82406=CARTESIAN_POINT('Ctrl Pts',(187.020322757229,31.9488468045685,0.));
#82407=CARTESIAN_POINT('Ctrl Pts',(187.697855441439,31.854052831669,0.));
#82408=CARTESIAN_POINT('Ctrl Pts',(187.697855441439,31.854052831669,31.854052831669));
#82409=CARTESIAN_POINT('Ctrl Pts',(187.697855441439,0.,31.854052831669));
#82410=CARTESIAN_POINT('Ctrl Pts',(187.697855441439,-31.854052831669,31.854052831669));
#82411=CARTESIAN_POINT('Ctrl Pts',(187.697855441439,-31.854052831669,0.));
#82412=CARTESIAN_POINT('Ctrl Pts',(187.697855441439,-31.854052831669,-31.854052831669));
#82413=CARTESIAN_POINT('Ctrl Pts',(187.697855441439,0.,-31.854052831669));
#82414=CARTESIAN_POINT('Ctrl Pts',(187.697855441439,31.854052831669,-31.854052831669));
#82415=CARTESIAN_POINT('Ctrl Pts',(187.697855441439,31.854052831669,0.));
#82416=CARTESIAN_POINT('Ctrl Pts',(188.37888266216,31.5613864248805,0.));
#82417=CARTESIAN_POINT('Ctrl Pts',(188.37888266216,31.5613864248805,31.5613864248805));
#82418=CARTESIAN_POINT('Ctrl Pts',(188.37888266216,0.,31.5613864248805));
#82419=CARTESIAN_POINT('Ctrl Pts',(188.37888266216,-31.5613864248805,31.5613864248805));
#82420=CARTESIAN_POINT('Ctrl Pts',(188.37888266216,-31.5613864248805,0.));
#82421=CARTESIAN_POINT('Ctrl Pts',(188.37888266216,-31.5613864248805,-31.5613864248805));
#82422=CARTESIAN_POINT('Ctrl Pts',(188.37888266216,0.,-31.5613864248805));
#82423=CARTESIAN_POINT('Ctrl Pts',(188.37888266216,31.5613864248805,-31.5613864248805));
#82424=CARTESIAN_POINT('Ctrl Pts',(188.37888266216,31.5613864248805,0.));
#82425=CARTESIAN_POINT('Ctrl Pts',(189.064450793941,31.0831127500011,0.));
#82426=CARTESIAN_POINT('Ctrl Pts',(189.064450793941,31.0831127500011,31.0831127500011));
#82427=CARTESIAN_POINT('Ctrl Pts',(189.064450793941,0.,31.0831127500011));
#82428=CARTESIAN_POINT('Ctrl Pts',(189.064450793941,-31.0831127500011,31.0831127500011));
#82429=CARTESIAN_POINT('Ctrl Pts',(189.064450793941,-31.0831127500011,0.));
#82430=CARTESIAN_POINT('Ctrl Pts',(189.064450793941,-31.0831127500011,-31.0831127500011));
#82431=CARTESIAN_POINT('Ctrl Pts',(189.064450793941,0.,-31.0831127500011));
#82432=CARTESIAN_POINT('Ctrl Pts',(189.064450793941,31.0831127500011,-31.0831127500011));
#82433=CARTESIAN_POINT('Ctrl Pts',(189.064450793941,31.0831127500011,0.));
#82434=CARTESIAN_POINT('Ctrl Pts',(189.75112407993,30.4394160167154,0.));
#82435=CARTESIAN_POINT('Ctrl Pts',(189.75112407993,30.4394160167154,30.4394160167154));
#82436=CARTESIAN_POINT('Ctrl Pts',(189.75112407993,0.,30.4394160167154));
#82437=CARTESIAN_POINT('Ctrl Pts',(189.75112407993,-30.4394160167154,30.4394160167154));
#82438=CARTESIAN_POINT('Ctrl Pts',(189.75112407993,-30.4394160167154,0.));
#82439=CARTESIAN_POINT('Ctrl Pts',(189.75112407993,-30.4394160167154,-30.4394160167154));
#82440=CARTESIAN_POINT('Ctrl Pts',(189.75112407993,0.,-30.4394160167154));
#82441=CARTESIAN_POINT('Ctrl Pts',(189.75112407993,30.4394160167154,-30.4394160167154));
#82442=CARTESIAN_POINT('Ctrl Pts',(189.75112407993,30.4394160167154,0.));
#82443=CARTESIAN_POINT('Ctrl Pts',(190.433084076035,29.6594255092613,0.));
#82444=CARTESIAN_POINT('Ctrl Pts',(190.433084076035,29.6594255092613,29.6594255092613));
#82445=CARTESIAN_POINT('Ctrl Pts',(190.433084076035,0.,29.6594255092613));
#82446=CARTESIAN_POINT('Ctrl Pts',(190.433084076035,-29.6594255092613,29.6594255092613));
#82447=CARTESIAN_POINT('Ctrl Pts',(190.433084076035,-29.6594255092613,0.));
#82448=CARTESIAN_POINT('Ctrl Pts',(190.433084076035,-29.6594255092613,-29.6594255092613));
#82449=CARTESIAN_POINT('Ctrl Pts',(190.433084076035,0.,-29.6594255092613));
#82450=CARTESIAN_POINT('Ctrl Pts',(190.433084076035,29.6594255092613,-29.6594255092613));
#82451=CARTESIAN_POINT('Ctrl Pts',(190.433084076035,29.6594255092613,0.));
#82452=CARTESIAN_POINT('Ctrl Pts',(191.103572014169,28.781420151568,0.));
#82453=CARTESIAN_POINT('Ctrl Pts',(191.103572014169,28.781420151568,28.781420151568));
#82454=CARTESIAN_POINT('Ctrl Pts',(191.103572014169,0.,28.781420151568));
#82455=CARTESIAN_POINT('Ctrl Pts',(191.103572014169,-28.781420151568,28.781420151568));
#82456=CARTESIAN_POINT('Ctrl Pts',(191.103572014169,-28.781420151568,0.));
#82457=CARTESIAN_POINT('Ctrl Pts',(191.103572014169,-28.781420151568,-28.781420151568));
#82458=CARTESIAN_POINT('Ctrl Pts',(191.103572014169,0.,-28.781420151568));
#82459=CARTESIAN_POINT('Ctrl Pts',(191.103572014169,28.781420151568,-28.781420151568));
#82460=CARTESIAN_POINT('Ctrl Pts',(191.103572014169,28.781420151568,0.));
#82461=CARTESIAN_POINT('Ctrl Pts',(191.756675094258,27.853709335318,0.));
#82462=CARTESIAN_POINT('Ctrl Pts',(191.756675094258,27.853709335318,27.853709335318));
#82463=CARTESIAN_POINT('Ctrl Pts',(191.756675094258,0.,27.853709335318));
#82464=CARTESIAN_POINT('Ctrl Pts',(191.756675094258,-27.853709335318,27.853709335318));
#82465=CARTESIAN_POINT('Ctrl Pts',(191.756675094258,-27.853709335318,0.));
#82466=CARTESIAN_POINT('Ctrl Pts',(191.756675094258,-27.853709335318,-27.853709335318));
#82467=CARTESIAN_POINT('Ctrl Pts',(191.756675094258,0.,-27.853709335318));
#82468=CARTESIAN_POINT('Ctrl Pts',(191.756675094258,27.853709335318,-27.853709335318));
#82469=CARTESIAN_POINT('Ctrl Pts',(191.756675094258,27.853709335318,0.));
#82470=CARTESIAN_POINT('Ctrl Pts',(192.388791155139,26.9344733292055,0.));
#82471=CARTESIAN_POINT('Ctrl Pts',(192.388791155139,26.9344733292055,26.9344733292055));
#82472=CARTESIAN_POINT('Ctrl Pts',(192.388791155139,0.,26.9344733292055));
#82473=CARTESIAN_POINT('Ctrl Pts',(192.388791155139,-26.9344733292055,26.9344733292055));
#82474=CARTESIAN_POINT('Ctrl Pts',(192.388791155139,-26.9344733292055,0.));
#82475=CARTESIAN_POINT('Ctrl Pts',(192.388791155139,-26.9344733292055,-26.9344733292055));
#82476=CARTESIAN_POINT('Ctrl Pts',(192.388791155139,0.,-26.9344733292055));
#82477=CARTESIAN_POINT('Ctrl Pts',(192.388791155139,26.9344733292055,-26.9344733292055));
#82478=CARTESIAN_POINT('Ctrl Pts',(192.388791155139,26.9344733292055,0.));
#82479=CARTESIAN_POINT('Ctrl Pts',(193.000672363666,26.0939712858825,0.));
#82480=CARTESIAN_POINT('Ctrl Pts',(193.000672363666,26.0939712858825,26.0939712858825));
#82481=CARTESIAN_POINT('Ctrl Pts',(193.000672363666,0.,26.0939712858825));
#82482=CARTESIAN_POINT('Ctrl Pts',(193.000672363666,-26.0939712858825,26.0939712858825));
#82483=CARTESIAN_POINT('Ctrl Pts',(193.000672363666,-26.0939712858825,0.));
#82484=CARTESIAN_POINT('Ctrl Pts',(193.000672363666,-26.0939712858825,-26.0939712858825));
#82485=CARTESIAN_POINT('Ctrl Pts',(193.000672363666,0.,-26.0939712858825));
#82486=CARTESIAN_POINT('Ctrl Pts',(193.000672363666,26.0939712858825,-26.0939712858825));
#82487=CARTESIAN_POINT('Ctrl Pts',(193.000672363666,26.0939712858825,0.));
#82488=CARTESIAN_POINT('Ctrl Pts',(193.597176293606,25.4069487182106,0.));
#82489=CARTESIAN_POINT('Ctrl Pts',(193.597176293606,25.4069487182106,25.4069487182106));
#82490=CARTESIAN_POINT('Ctrl Pts',(193.597176293606,0.,25.4069487182106));
#82491=CARTESIAN_POINT('Ctrl Pts',(193.597176293606,-25.4069487182106,25.4069487182106));
#82492=CARTESIAN_POINT('Ctrl Pts',(193.597176293606,-25.4069487182106,0.));
#82493=CARTESIAN_POINT('Ctrl Pts',(193.597176293606,-25.4069487182106,-25.4069487182106));
#82494=CARTESIAN_POINT('Ctrl Pts',(193.597176293606,0.,-25.4069487182106));
#82495=CARTESIAN_POINT('Ctrl Pts',(193.597176293606,25.4069487182106,-25.4069487182106));
#82496=CARTESIAN_POINT('Ctrl Pts',(193.597176293606,25.4069487182106,0.));
#82497=CARTESIAN_POINT('Ctrl Pts',(194.185626322862,24.9394496497274,0.));
#82498=CARTESIAN_POINT('Ctrl Pts',(194.185626322862,24.9394496497274,24.9394496497274));
#82499=CARTESIAN_POINT('Ctrl Pts',(194.185626322862,0.,24.9394496497274));
#82500=CARTESIAN_POINT('Ctrl Pts',(194.185626322862,-24.9394496497274,24.9394496497274));
#82501=CARTESIAN_POINT('Ctrl Pts',(194.185626322862,-24.9394496497274,0.));
#82502=CARTESIAN_POINT('Ctrl Pts',(194.185626322862,-24.9394496497274,-24.9394496497274));
#82503=CARTESIAN_POINT('Ctrl Pts',(194.185626322862,0.,-24.9394496497274));
#82504=CARTESIAN_POINT('Ctrl Pts',(194.185626322862,24.9394496497274,-24.9394496497274));
#82505=CARTESIAN_POINT('Ctrl Pts',(194.185626322862,24.9394496497274,0.));
#82506=CARTESIAN_POINT('Ctrl Pts',(194.774568374152,24.7365253484543,0.));
#82507=CARTESIAN_POINT('Ctrl Pts',(194.774568374152,24.7365253484542,24.7365253484542));
#82508=CARTESIAN_POINT('Ctrl Pts',(194.774568374152,0.,24.7365253484543));
#82509=CARTESIAN_POINT('Ctrl Pts',(194.774568374152,-24.7365253484542,24.7365253484542));
#82510=CARTESIAN_POINT('Ctrl Pts',(194.774568374152,-24.7365253484543,0.));
#82511=CARTESIAN_POINT('Ctrl Pts',(194.774568374152,-24.7365253484542,-24.7365253484542));
#82512=CARTESIAN_POINT('Ctrl Pts',(194.774568374152,0.,-24.7365253484543));
#82513=CARTESIAN_POINT('Ctrl Pts',(194.774568374152,24.7365253484542,-24.7365253484542));
#82514=CARTESIAN_POINT('Ctrl Pts',(194.774568374152,24.7365253484543,0.));
#82515=CARTESIAN_POINT('Ctrl Pts',(195.372421781966,24.8112917102097,0.));
#82516=CARTESIAN_POINT('Ctrl Pts',(195.372421781966,24.8112917102097,24.8112917102097));
#82517=CARTESIAN_POINT('Ctrl Pts',(195.372421781966,0.,24.8112917102097));
#82518=CARTESIAN_POINT('Ctrl Pts',(195.372421781966,-24.8112917102097,24.8112917102097));
#82519=CARTESIAN_POINT('Ctrl Pts',(195.372421781966,-24.8112917102097,0.));
#82520=CARTESIAN_POINT('Ctrl Pts',(195.372421781966,-24.8112917102097,-24.8112917102097));
#82521=CARTESIAN_POINT('Ctrl Pts',(195.372421781966,0.,-24.8112917102097));
#82522=CARTESIAN_POINT('Ctrl Pts',(195.372421781966,24.8112917102097,-24.8112917102097));
#82523=CARTESIAN_POINT('Ctrl Pts',(195.372421781966,24.8112917102097,0.));
#82524=CARTESIAN_POINT('Ctrl Pts',(195.986035381944,25.1290290983464,0.));
#82525=CARTESIAN_POINT('Ctrl Pts',(195.986035381944,25.1290290983464,25.1290290983464));
#82526=CARTESIAN_POINT('Ctrl Pts',(195.986035381944,0.,25.1290290983464));
#82527=CARTESIAN_POINT('Ctrl Pts',(195.986035381944,-25.1290290983464,25.1290290983464));
#82528=CARTESIAN_POINT('Ctrl Pts',(195.986035381944,-25.1290290983464,0.));
#82529=CARTESIAN_POINT('Ctrl Pts',(195.986035381944,-25.1290290983464,-25.1290290983464));
#82530=CARTESIAN_POINT('Ctrl Pts',(195.986035381944,0.,-25.1290290983464));
#82531=CARTESIAN_POINT('Ctrl Pts',(195.986035381944,25.1290290983464,-25.1290290983464));
#82532=CARTESIAN_POINT('Ctrl Pts',(195.986035381944,25.1290290983464,0.));
#82533=CARTESIAN_POINT('Ctrl Pts',(196.61996014565,25.6142225395129,0.));
#82534=CARTESIAN_POINT('Ctrl Pts',(196.61996014565,25.6142225395129,25.6142225395129));
#82535=CARTESIAN_POINT('Ctrl Pts',(196.61996014565,0.,25.6142225395129));
#82536=CARTESIAN_POINT('Ctrl Pts',(196.61996014565,-25.6142225395129,25.6142225395129));
#82537=CARTESIAN_POINT('Ctrl Pts',(196.61996014565,-25.6142225395129,0.));
#82538=CARTESIAN_POINT('Ctrl Pts',(196.61996014565,-25.6142225395129,-25.6142225395129));
#82539=CARTESIAN_POINT('Ctrl Pts',(196.61996014565,0.,-25.6142225395129));
#82540=CARTESIAN_POINT('Ctrl Pts',(196.61996014565,25.6142225395129,-25.6142225395129));
#82541=CARTESIAN_POINT('Ctrl Pts',(196.61996014565,25.6142225395129,0.));
#82542=CARTESIAN_POINT('Ctrl Pts',(197.27617886607,26.1710294150248,0.));
#82543=CARTESIAN_POINT('Ctrl Pts',(197.27617886607,26.1710294150248,26.1710294150248));
#82544=CARTESIAN_POINT('Ctrl Pts',(197.27617886607,0.,26.1710294150248));
#82545=CARTESIAN_POINT('Ctrl Pts',(197.27617886607,-26.1710294150248,26.1710294150248));
#82546=CARTESIAN_POINT('Ctrl Pts',(197.27617886607,-26.1710294150248,0.));
#82547=CARTESIAN_POINT('Ctrl Pts',(197.27617886607,-26.1710294150248,-26.1710294150248));
#82548=CARTESIAN_POINT('Ctrl Pts',(197.27617886607,0.,-26.1710294150248));
#82549=CARTESIAN_POINT('Ctrl Pts',(197.27617886607,26.1710294150248,-26.1710294150248));
#82550=CARTESIAN_POINT('Ctrl Pts',(197.27617886607,26.1710294150248,0.));
#82551=CARTESIAN_POINT('Ctrl Pts',(197.953680886587,26.6997761508392,0.));
#82552=CARTESIAN_POINT('Ctrl Pts',(197.953680886587,26.6997761508392,26.6997761508392));
#82553=CARTESIAN_POINT('Ctrl Pts',(197.953680886587,0.,26.6997761508392));
#82554=CARTESIAN_POINT('Ctrl Pts',(197.953680886587,-26.6997761508392,26.6997761508392));
#82555=CARTESIAN_POINT('Ctrl Pts',(197.953680886587,-26.6997761508392,0.));
#82556=CARTESIAN_POINT('Ctrl Pts',(197.953680886587,-26.6997761508392,-26.6997761508392));
#82557=CARTESIAN_POINT('Ctrl Pts',(197.953680886587,0.,-26.6997761508392));
#82558=CARTESIAN_POINT('Ctrl Pts',(197.953680886587,26.6997761508392,-26.6997761508392));
#82559=CARTESIAN_POINT('Ctrl Pts',(197.953680886587,26.6997761508392,0.));
#82560=CARTESIAN_POINT('Ctrl Pts',(198.64812240998,27.1147192657497,0.));
#82561=CARTESIAN_POINT('Ctrl Pts',(198.64812240998,27.1147192657497,27.1147192657497));
#82562=CARTESIAN_POINT('Ctrl Pts',(198.64812240998,0.,27.1147192657497));
#82563=CARTESIAN_POINT('Ctrl Pts',(198.64812240998,-27.1147192657497,27.1147192657497));
#82564=CARTESIAN_POINT('Ctrl Pts',(198.64812240998,-27.1147192657497,0.));
#82565=CARTESIAN_POINT('Ctrl Pts',(198.64812240998,-27.1147192657497,-27.1147192657497));
#82566=CARTESIAN_POINT('Ctrl Pts',(198.64812240998,0.,-27.1147192657497));
#82567=CARTESIAN_POINT('Ctrl Pts',(198.64812240998,27.1147192657497,-27.1147192657497));
#82568=CARTESIAN_POINT('Ctrl Pts',(198.64812240998,27.1147192657497,0.));
#82569=CARTESIAN_POINT('Ctrl Pts',(199.351380905309,27.3622787234429,0.));
#82570=CARTESIAN_POINT('Ctrl Pts',(199.351380905309,27.3622787234429,27.3622787234429));
#82571=CARTESIAN_POINT('Ctrl Pts',(199.351380905309,0.,27.3622787234429));
#82572=CARTESIAN_POINT('Ctrl Pts',(199.351380905309,-27.3622787234429,27.3622787234429));
#82573=CARTESIAN_POINT('Ctrl Pts',(199.351380905309,-27.3622787234429,0.));
#82574=CARTESIAN_POINT('Ctrl Pts',(199.351380905309,-27.3622787234429,-27.3622787234429));
#82575=CARTESIAN_POINT('Ctrl Pts',(199.351380905309,0.,-27.3622787234429));
#82576=CARTESIAN_POINT('Ctrl Pts',(199.351380905309,27.3622787234429,-27.3622787234429));
#82577=CARTESIAN_POINT('Ctrl Pts',(199.351380905309,27.3622787234429,0.));
#82578=CARTESIAN_POINT('Ctrl Pts',(200.052580368893,27.4153142520686,0.));
#82579=CARTESIAN_POINT('Ctrl Pts',(200.052580368893,27.4153142520686,27.4153142520686));
#82580=CARTESIAN_POINT('Ctrl Pts',(200.052580368893,0.,27.4153142520686));
#82581=CARTESIAN_POINT('Ctrl Pts',(200.052580368893,-27.4153142520686,27.4153142520686));
#82582=CARTESIAN_POINT('Ctrl Pts',(200.052580368893,-27.4153142520686,0.));
#82583=CARTESIAN_POINT('Ctrl Pts',(200.052580368893,-27.4153142520686,-27.4153142520686));
#82584=CARTESIAN_POINT('Ctrl Pts',(200.052580368893,0.,-27.4153142520686));
#82585=CARTESIAN_POINT('Ctrl Pts',(200.052580368893,27.4153142520686,-27.4153142520686));
#82586=CARTESIAN_POINT('Ctrl Pts',(200.052580368893,27.4153142520686,0.));
#82587=CARTESIAN_POINT('Ctrl Pts',(200.739177478596,27.2655121051523,0.));
#82588=CARTESIAN_POINT('Ctrl Pts',(200.739177478596,27.2655121051522,27.2655121051522));
#82589=CARTESIAN_POINT('Ctrl Pts',(200.739177478596,0.,27.2655121051523));
#82590=CARTESIAN_POINT('Ctrl Pts',(200.739177478596,-27.2655121051522,27.2655121051522));
#82591=CARTESIAN_POINT('Ctrl Pts',(200.739177478596,-27.2655121051523,0.));
#82592=CARTESIAN_POINT('Ctrl Pts',(200.739177478596,-27.2655121051522,-27.2655121051522));
#82593=CARTESIAN_POINT('Ctrl Pts',(200.739177478596,0.,-27.2655121051523));
#82594=CARTESIAN_POINT('Ctrl Pts',(200.739177478596,27.2655121051522,-27.2655121051522));
#82595=CARTESIAN_POINT('Ctrl Pts',(200.739177478596,27.2655121051523,0.));
#82596=CARTESIAN_POINT('Ctrl Pts',(201.39806187553,26.9171117141031,0.));
#82597=CARTESIAN_POINT('Ctrl Pts',(201.39806187553,26.9171117141031,26.9171117141031));
#82598=CARTESIAN_POINT('Ctrl Pts',(201.39806187553,0.,26.9171117141031));
#82599=CARTESIAN_POINT('Ctrl Pts',(201.39806187553,-26.9171117141031,26.9171117141031));
#82600=CARTESIAN_POINT('Ctrl Pts',(201.39806187553,-26.9171117141031,0.));
#82601=CARTESIAN_POINT('Ctrl Pts',(201.39806187553,-26.9171117141031,-26.9171117141031));
#82602=CARTESIAN_POINT('Ctrl Pts',(201.39806187553,0.,-26.9171117141031));
#82603=CARTESIAN_POINT('Ctrl Pts',(201.39806187553,26.9171117141031,-26.9171117141031));
#82604=CARTESIAN_POINT('Ctrl Pts',(201.39806187553,26.9171117141031,0.));
#82605=CARTESIAN_POINT('Ctrl Pts',(202.016556766229,26.3785672681198,0.));
#82606=CARTESIAN_POINT('Ctrl Pts',(202.016556766229,26.3785672681198,26.3785672681198));
#82607=CARTESIAN_POINT('Ctrl Pts',(202.016556766229,0.,26.3785672681198));
#82608=CARTESIAN_POINT('Ctrl Pts',(202.016556766229,-26.3785672681198,26.3785672681198));
#82609=CARTESIAN_POINT('Ctrl Pts',(202.016556766229,-26.3785672681198,0.));
#82610=CARTESIAN_POINT('Ctrl Pts',(202.016556766229,-26.3785672681198,-26.3785672681198));
#82611=CARTESIAN_POINT('Ctrl Pts',(202.016556766229,0.,-26.3785672681198));
#82612=CARTESIAN_POINT('Ctrl Pts',(202.016556766229,26.3785672681198,-26.3785672681198));
#82613=CARTESIAN_POINT('Ctrl Pts',(202.016556766229,26.3785672681198,0.));
#82614=CARTESIAN_POINT('Ctrl Pts',(202.583897300149,25.6620387985065,0.));
#82615=CARTESIAN_POINT('Ctrl Pts',(202.583897300149,25.6620387985065,25.6620387985065));
#82616=CARTESIAN_POINT('Ctrl Pts',(202.583897300149,0.,25.6620387985065));
#82617=CARTESIAN_POINT('Ctrl Pts',(202.583897300149,-25.6620387985065,25.6620387985065));
#82618=CARTESIAN_POINT('Ctrl Pts',(202.583897300149,-25.6620387985065,0.));
#82619=CARTESIAN_POINT('Ctrl Pts',(202.583897300149,-25.6620387985065,-25.6620387985065));
#82620=CARTESIAN_POINT('Ctrl Pts',(202.583897300149,0.,-25.6620387985065));
#82621=CARTESIAN_POINT('Ctrl Pts',(202.583897300149,25.6620387985065,-25.6620387985065));
#82622=CARTESIAN_POINT('Ctrl Pts',(202.583897300149,25.6620387985065,0.));
#82623=CARTESIAN_POINT('Ctrl Pts',(203.093076162889,24.7880448411392,0.));
#82624=CARTESIAN_POINT('Ctrl Pts',(203.093076162889,24.7880448411392,24.7880448411392));
#82625=CARTESIAN_POINT('Ctrl Pts',(203.093076162889,0.,24.7880448411392));
#82626=CARTESIAN_POINT('Ctrl Pts',(203.093076162889,-24.7880448411392,24.7880448411392));
#82627=CARTESIAN_POINT('Ctrl Pts',(203.093076162889,-24.7880448411392,0.));
#82628=CARTESIAN_POINT('Ctrl Pts',(203.093076162889,-24.7880448411392,-24.7880448411392));
#82629=CARTESIAN_POINT('Ctrl Pts',(203.093076162889,0.,-24.7880448411392));
#82630=CARTESIAN_POINT('Ctrl Pts',(203.093076162889,24.7880448411392,-24.7880448411392));
#82631=CARTESIAN_POINT('Ctrl Pts',(203.093076162889,24.7880448411392,0.));
#82632=CARTESIAN_POINT('Ctrl Pts',(203.542511863345,23.7884093162236,0.));
#82633=CARTESIAN_POINT('Ctrl Pts',(203.542511863345,23.7884093162236,23.7884093162236));
#82634=CARTESIAN_POINT('Ctrl Pts',(203.542511863345,0.,23.7884093162236));
#82635=CARTESIAN_POINT('Ctrl Pts',(203.542511863345,-23.7884093162236,23.7884093162236));
#82636=CARTESIAN_POINT('Ctrl Pts',(203.542511863345,-23.7884093162236,0.));
#82637=CARTESIAN_POINT('Ctrl Pts',(203.542511863345,-23.7884093162236,-23.7884093162236));
#82638=CARTESIAN_POINT('Ctrl Pts',(203.542511863345,0.,-23.7884093162236));
#82639=CARTESIAN_POINT('Ctrl Pts',(203.542511863345,23.7884093162236,-23.7884093162236));
#82640=CARTESIAN_POINT('Ctrl Pts',(203.542511863345,23.7884093162236,0.));
#82641=CARTESIAN_POINT('Ctrl Pts',(203.937951189067,22.7103152246357,0.));
#82642=CARTESIAN_POINT('Ctrl Pts',(203.937951189067,22.7103152246357,22.7103152246357));
#82643=CARTESIAN_POINT('Ctrl Pts',(203.937951189067,0.,22.7103152246357));
#82644=CARTESIAN_POINT('Ctrl Pts',(203.937951189067,-22.7103152246357,22.7103152246357));
#82645=CARTESIAN_POINT('Ctrl Pts',(203.937951189067,-22.7103152246357,0.));
#82646=CARTESIAN_POINT('Ctrl Pts',(203.937951189067,-22.7103152246357,-22.7103152246357));
#82647=CARTESIAN_POINT('Ctrl Pts',(203.937951189067,0.,-22.7103152246357));
#82648=CARTESIAN_POINT('Ctrl Pts',(203.937951189067,22.7103152246357,-22.7103152246357));
#82649=CARTESIAN_POINT('Ctrl Pts',(203.937951189067,22.7103152246357,0.));
#82650=CARTESIAN_POINT('Ctrl Pts',(204.293916519169,21.6189881673319,0.));
#82651=CARTESIAN_POINT('Ctrl Pts',(204.293916519169,21.6189881673319,21.6189881673319));
#82652=CARTESIAN_POINT('Ctrl Pts',(204.293916519169,0.,21.6189881673319));
#82653=CARTESIAN_POINT('Ctrl Pts',(204.293916519169,-21.6189881673319,21.6189881673319));
#82654=CARTESIAN_POINT('Ctrl Pts',(204.293916519169,-21.6189881673319,0.));
#82655=CARTESIAN_POINT('Ctrl Pts',(204.293916519169,-21.6189881673319,-21.6189881673319));
#82656=CARTESIAN_POINT('Ctrl Pts',(204.293916519169,0.,-21.6189881673319));
#82657=CARTESIAN_POINT('Ctrl Pts',(204.293916519169,21.6189881673319,-21.6189881673319));
#82658=CARTESIAN_POINT('Ctrl Pts',(204.293916519169,21.6189881673319,0.));
#82659=CARTESIAN_POINT('Ctrl Pts',(204.636303489551,20.6033665580493,0.));
#82660=CARTESIAN_POINT('Ctrl Pts',(204.636303489551,20.6033665580493,20.6033665580493));
#82661=CARTESIAN_POINT('Ctrl Pts',(204.636303489551,0.,20.6033665580493));
#82662=CARTESIAN_POINT('Ctrl Pts',(204.636303489551,-20.6033665580493,20.6033665580493));
#82663=CARTESIAN_POINT('Ctrl Pts',(204.636303489551,-20.6033665580493,0.));
#82664=CARTESIAN_POINT('Ctrl Pts',(204.636303489551,-20.6033665580493,-20.6033665580493));
#82665=CARTESIAN_POINT('Ctrl Pts',(204.636303489551,0.,-20.6033665580493));
#82666=CARTESIAN_POINT('Ctrl Pts',(204.636303489551,20.6033665580493,-20.6033665580493));
#82667=CARTESIAN_POINT('Ctrl Pts',(204.636303489551,20.6033665580493,0.));
#82668=CARTESIAN_POINT('Ctrl Pts',(204.996948764239,19.7615251622739,0.));
#82669=CARTESIAN_POINT('Ctrl Pts',(204.996948764239,19.7615251622739,19.7615251622739));
#82670=CARTESIAN_POINT('Ctrl Pts',(204.996948764239,0.,19.7615251622739));
#82671=CARTESIAN_POINT('Ctrl Pts',(204.996948764239,-19.7615251622739,19.7615251622739));
#82672=CARTESIAN_POINT('Ctrl Pts',(204.996948764239,-19.7615251622739,0.));
#82673=CARTESIAN_POINT('Ctrl Pts',(204.996948764239,-19.7615251622739,-19.7615251622739));
#82674=CARTESIAN_POINT('Ctrl Pts',(204.996948764239,0.,-19.7615251622739));
#82675=CARTESIAN_POINT('Ctrl Pts',(204.996948764239,19.7615251622739,-19.7615251622739));
#82676=CARTESIAN_POINT('Ctrl Pts',(204.996948764239,19.7615251622739,0.));
#82677=CARTESIAN_POINT('Ctrl Pts',(205.406561032152,19.1819945300443,0.));
#82678=CARTESIAN_POINT('Ctrl Pts',(205.406561032152,19.1819945300443,19.1819945300443));
#82679=CARTESIAN_POINT('Ctrl Pts',(205.406561032152,0.,19.1819945300443));
#82680=CARTESIAN_POINT('Ctrl Pts',(205.406561032152,-19.1819945300443,19.1819945300443));
#82681=CARTESIAN_POINT('Ctrl Pts',(205.406561032152,-19.1819945300443,0.));
#82682=CARTESIAN_POINT('Ctrl Pts',(205.406561032152,-19.1819945300443,-19.1819945300443));
#82683=CARTESIAN_POINT('Ctrl Pts',(205.406561032152,0.,-19.1819945300443));
#82684=CARTESIAN_POINT('Ctrl Pts',(205.406561032152,19.1819945300443,-19.1819945300443));
#82685=CARTESIAN_POINT('Ctrl Pts',(205.406561032152,19.1819945300443,0.));
#82686=CARTESIAN_POINT('Ctrl Pts',(205.887941237232,18.9257935294742,0.));
#82687=CARTESIAN_POINT('Ctrl Pts',(205.887941237232,18.9257935294742,18.9257935294742));
#82688=CARTESIAN_POINT('Ctrl Pts',(205.887941237232,0.,18.9257935294742));
#82689=CARTESIAN_POINT('Ctrl Pts',(205.887941237232,-18.9257935294742,18.9257935294742));
#82690=CARTESIAN_POINT('Ctrl Pts',(205.887941237232,-18.9257935294742,0.));
#82691=CARTESIAN_POINT('Ctrl Pts',(205.887941237232,-18.9257935294742,-18.9257935294742));
#82692=CARTESIAN_POINT('Ctrl Pts',(205.887941237232,0.,-18.9257935294742));
#82693=CARTESIAN_POINT('Ctrl Pts',(205.887941237232,18.9257935294742,-18.9257935294742));
#82694=CARTESIAN_POINT('Ctrl Pts',(205.887941237232,18.9257935294742,0.));
#82695=CARTESIAN_POINT('Ctrl Pts',(206.449692896782,19.0096950757953,0.));
#82696=CARTESIAN_POINT('Ctrl Pts',(206.449692896782,19.0096950757953,19.0096950757953));
#82697=CARTESIAN_POINT('Ctrl Pts',(206.449692896782,0.,19.0096950757953));
#82698=CARTESIAN_POINT('Ctrl Pts',(206.449692896782,-19.0096950757953,19.0096950757953));
#82699=CARTESIAN_POINT('Ctrl Pts',(206.449692896782,-19.0096950757953,0.));
#82700=CARTESIAN_POINT('Ctrl Pts',(206.449692896782,-19.0096950757953,-19.0096950757953));
#82701=CARTESIAN_POINT('Ctrl Pts',(206.449692896782,0.,-19.0096950757953));
#82702=CARTESIAN_POINT('Ctrl Pts',(206.449692896782,19.0096950757953,-19.0096950757953));
#82703=CARTESIAN_POINT('Ctrl Pts',(206.449692896782,19.0096950757953,0.));
#82704=CARTESIAN_POINT('Ctrl Pts',(207.078090239928,19.3848418671143,0.));
#82705=CARTESIAN_POINT('Ctrl Pts',(207.078090239928,19.3848418671143,19.3848418671143));
#82706=CARTESIAN_POINT('Ctrl Pts',(207.078090239928,0.,19.3848418671143));
#82707=CARTESIAN_POINT('Ctrl Pts',(207.078090239928,-19.3848418671143,19.3848418671143));
#82708=CARTESIAN_POINT('Ctrl Pts',(207.078090239928,-19.3848418671143,0.));
#82709=CARTESIAN_POINT('Ctrl Pts',(207.078090239928,-19.3848418671143,-19.3848418671143));
#82710=CARTESIAN_POINT('Ctrl Pts',(207.078090239928,0.,-19.3848418671143));
#82711=CARTESIAN_POINT('Ctrl Pts',(207.078090239928,19.3848418671143,-19.3848418671143));
#82712=CARTESIAN_POINT('Ctrl Pts',(207.078090239928,19.3848418671143,0.));
#82713=CARTESIAN_POINT('Ctrl Pts',(207.744015652215,19.9532689458847,0.));
#82714=CARTESIAN_POINT('Ctrl Pts',(207.744015652215,19.9532689458847,19.9532689458847));
#82715=CARTESIAN_POINT('Ctrl Pts',(207.744015652215,0.,19.9532689458847));
#82716=CARTESIAN_POINT('Ctrl Pts',(207.744015652215,-19.9532689458847,19.9532689458847));
#82717=CARTESIAN_POINT('Ctrl Pts',(207.744015652215,-19.9532689458847,0.));
#82718=CARTESIAN_POINT('Ctrl Pts',(207.744015652215,-19.9532689458847,-19.9532689458847));
#82719=CARTESIAN_POINT('Ctrl Pts',(207.744015652215,0.,-19.9532689458847));
#82720=CARTESIAN_POINT('Ctrl Pts',(207.744015652215,19.9532689458847,-19.9532689458847));
#82721=CARTESIAN_POINT('Ctrl Pts',(207.744015652215,19.9532689458847,0.));
#82722=CARTESIAN_POINT('Ctrl Pts',(208.412972675131,20.5920992378761,0.));
#82723=CARTESIAN_POINT('Ctrl Pts',(208.412972675131,20.5920992378761,20.5920992378761));
#82724=CARTESIAN_POINT('Ctrl Pts',(208.412972675131,0.,20.5920992378761));
#82725=CARTESIAN_POINT('Ctrl Pts',(208.412972675131,-20.5920992378761,20.5920992378761));
#82726=CARTESIAN_POINT('Ctrl Pts',(208.412972675131,-20.5920992378761,0.));
#82727=CARTESIAN_POINT('Ctrl Pts',(208.412972675131,-20.5920992378761,-20.5920992378761));
#82728=CARTESIAN_POINT('Ctrl Pts',(208.412972675131,0.,-20.5920992378761));
#82729=CARTESIAN_POINT('Ctrl Pts',(208.412972675131,20.5920992378761,-20.5920992378761));
#82730=CARTESIAN_POINT('Ctrl Pts',(208.412972675131,20.5920992378761,0.));
#82731=CARTESIAN_POINT('Ctrl Pts',(209.053888810014,21.1748081323919,0.));
#82732=CARTESIAN_POINT('Ctrl Pts',(209.053888810014,21.1748081323919,21.1748081323919));
#82733=CARTESIAN_POINT('Ctrl Pts',(209.053888810014,0.,21.1748081323919));
#82734=CARTESIAN_POINT('Ctrl Pts',(209.053888810014,-21.1748081323919,21.1748081323919));
#82735=CARTESIAN_POINT('Ctrl Pts',(209.053888810014,-21.1748081323919,0.));
#82736=CARTESIAN_POINT('Ctrl Pts',(209.053888810014,-21.1748081323919,-21.1748081323919));
#82737=CARTESIAN_POINT('Ctrl Pts',(209.053888810014,0.,-21.1748081323919));
#82738=CARTESIAN_POINT('Ctrl Pts',(209.053888810014,21.1748081323919,-21.1748081323919));
#82739=CARTESIAN_POINT('Ctrl Pts',(209.053888810014,21.1748081323919,0.));
#82740=CARTESIAN_POINT('Ctrl Pts',(209.648738296528,21.5942508361551,0.));
#82741=CARTESIAN_POINT('Ctrl Pts',(209.648738296528,21.5942508361551,21.5942508361551));
#82742=CARTESIAN_POINT('Ctrl Pts',(209.648738296528,0.,21.5942508361551));
#82743=CARTESIAN_POINT('Ctrl Pts',(209.648738296528,-21.5942508361551,21.5942508361551));
#82744=CARTESIAN_POINT('Ctrl Pts',(209.648738296528,-21.5942508361551,0.));
#82745=CARTESIAN_POINT('Ctrl Pts',(209.648738296528,-21.5942508361551,-21.5942508361551));
#82746=CARTESIAN_POINT('Ctrl Pts',(209.648738296528,0.,-21.5942508361551));
#82747=CARTESIAN_POINT('Ctrl Pts',(209.648738296528,21.5942508361551,-21.5942508361551));
#82748=CARTESIAN_POINT('Ctrl Pts',(209.648738296528,21.5942508361551,0.));
#82749=CARTESIAN_POINT('Ctrl Pts',(210.200918116375,21.7834157131811,0.));
#82750=CARTESIAN_POINT('Ctrl Pts',(210.200918116375,21.7834157131811,21.7834157131811));
#82751=CARTESIAN_POINT('Ctrl Pts',(210.200918116375,0.,21.7834157131811));
#82752=CARTESIAN_POINT('Ctrl Pts',(210.200918116375,-21.7834157131811,21.7834157131811));
#82753=CARTESIAN_POINT('Ctrl Pts',(210.200918116375,-21.7834157131811,0.));
#82754=CARTESIAN_POINT('Ctrl Pts',(210.200918116375,-21.7834157131811,-21.7834157131811));
#82755=CARTESIAN_POINT('Ctrl Pts',(210.200918116375,0.,-21.7834157131811));
#82756=CARTESIAN_POINT('Ctrl Pts',(210.200918116375,21.7834157131811,-21.7834157131811));
#82757=CARTESIAN_POINT('Ctrl Pts',(210.200918116375,21.7834157131811,0.));
#82758=CARTESIAN_POINT('Ctrl Pts',(210.725601433264,21.7102505096364,0.));
#82759=CARTESIAN_POINT('Ctrl Pts',(210.725601433264,21.7102505096364,21.7102505096364));
#82760=CARTESIAN_POINT('Ctrl Pts',(210.725601433264,0.,21.7102505096364));
#82761=CARTESIAN_POINT('Ctrl Pts',(210.725601433264,-21.7102505096364,21.7102505096364));
#82762=CARTESIAN_POINT('Ctrl Pts',(210.725601433264,-21.7102505096364,0.));
#82763=CARTESIAN_POINT('Ctrl Pts',(210.725601433264,-21.7102505096364,-21.7102505096364));
#82764=CARTESIAN_POINT('Ctrl Pts',(210.725601433264,0.,-21.7102505096364));
#82765=CARTESIAN_POINT('Ctrl Pts',(210.725601433264,21.7102505096364,-21.7102505096364));
#82766=CARTESIAN_POINT('Ctrl Pts',(210.725601433264,21.7102505096364,0.));
#82767=CARTESIAN_POINT('Ctrl Pts',(211.241810802359,21.3737042041621,0.));
#82768=CARTESIAN_POINT('Ctrl Pts',(211.241810802359,21.3737042041621,21.3737042041621));
#82769=CARTESIAN_POINT('Ctrl Pts',(211.241810802359,0.,21.3737042041621));
#82770=CARTESIAN_POINT('Ctrl Pts',(211.241810802359,-21.3737042041621,21.3737042041621));
#82771=CARTESIAN_POINT('Ctrl Pts',(211.241810802359,-21.3737042041621,0.));
#82772=CARTESIAN_POINT('Ctrl Pts',(211.241810802359,-21.3737042041621,-21.3737042041621));
#82773=CARTESIAN_POINT('Ctrl Pts',(211.241810802359,0.,-21.3737042041621));
#82774=CARTESIAN_POINT('Ctrl Pts',(211.241810802359,21.3737042041621,-21.3737042041621));
#82775=CARTESIAN_POINT('Ctrl Pts',(211.241810802359,21.3737042041621,0.));
#82776=CARTESIAN_POINT('Ctrl Pts',(211.762347225289,20.7998079091476,0.));
#82777=CARTESIAN_POINT('Ctrl Pts',(211.762347225289,20.7998079091476,20.7998079091476));
#82778=CARTESIAN_POINT('Ctrl Pts',(211.762347225289,0.,20.7998079091476));
#82779=CARTESIAN_POINT('Ctrl Pts',(211.762347225289,-20.7998079091476,20.7998079091476));
#82780=CARTESIAN_POINT('Ctrl Pts',(211.762347225289,-20.7998079091476,0.));
#82781=CARTESIAN_POINT('Ctrl Pts',(211.762347225289,-20.7998079091476,-20.7998079091476));
#82782=CARTESIAN_POINT('Ctrl Pts',(211.762347225289,0.,-20.7998079091476));
#82783=CARTESIAN_POINT('Ctrl Pts',(211.762347225289,20.7998079091476,-20.7998079091476));
#82784=CARTESIAN_POINT('Ctrl Pts',(211.762347225289,20.7998079091476,0.));
#82785=CARTESIAN_POINT('Ctrl Pts',(212.290210763329,20.0360509959614,0.));
#82786=CARTESIAN_POINT('Ctrl Pts',(212.290210763329,20.0360509959614,20.0360509959614));
#82787=CARTESIAN_POINT('Ctrl Pts',(212.290210763329,0.,20.0360509959614));
#82788=CARTESIAN_POINT('Ctrl Pts',(212.290210763329,-20.0360509959614,20.0360509959614));
#82789=CARTESIAN_POINT('Ctrl Pts',(212.290210763329,-20.0360509959614,0.));
#82790=CARTESIAN_POINT('Ctrl Pts',(212.290210763329,-20.0360509959614,-20.0360509959614));
#82791=CARTESIAN_POINT('Ctrl Pts',(212.290210763329,0.,-20.0360509959614));
#82792=CARTESIAN_POINT('Ctrl Pts',(212.290210763329,20.0360509959614,-20.0360509959614));
#82793=CARTESIAN_POINT('Ctrl Pts',(212.290210763329,20.0360509959614,0.));
#82794=CARTESIAN_POINT('Ctrl Pts',(212.822218578073,19.1433606114324,0.));
#82795=CARTESIAN_POINT('Ctrl Pts',(212.822218578073,19.1433606114324,19.1433606114324));
#82796=CARTESIAN_POINT('Ctrl Pts',(212.822218578073,0.,19.1433606114324));
#82797=CARTESIAN_POINT('Ctrl Pts',(212.822218578073,-19.1433606114324,19.1433606114324));
#82798=CARTESIAN_POINT('Ctrl Pts',(212.822218578073,-19.1433606114324,0.));
#82799=CARTESIAN_POINT('Ctrl Pts',(212.822218578073,-19.1433606114324,-19.1433606114324));
#82800=CARTESIAN_POINT('Ctrl Pts',(212.822218578073,0.,-19.1433606114324));
#82801=CARTESIAN_POINT('Ctrl Pts',(212.822218578073,19.1433606114324,-19.1433606114324));
#82802=CARTESIAN_POINT('Ctrl Pts',(212.822218578073,19.1433606114324,0.));
#82803=CARTESIAN_POINT('Ctrl Pts',(213.35072042915,18.1888571775611,0.));
#82804=CARTESIAN_POINT('Ctrl Pts',(213.35072042915,18.1888571775611,18.1888571775611));
#82805=CARTESIAN_POINT('Ctrl Pts',(213.35072042915,0.,18.1888571775611));
#82806=CARTESIAN_POINT('Ctrl Pts',(213.35072042915,-18.1888571775611,18.1888571775611));
#82807=CARTESIAN_POINT('Ctrl Pts',(213.35072042915,-18.1888571775611,0.));
#82808=CARTESIAN_POINT('Ctrl Pts',(213.35072042915,-18.1888571775611,-18.1888571775611));
#82809=CARTESIAN_POINT('Ctrl Pts',(213.35072042915,0.,-18.1888571775611));
#82810=CARTESIAN_POINT('Ctrl Pts',(213.35072042915,18.1888571775611,-18.1888571775611));
#82811=CARTESIAN_POINT('Ctrl Pts',(213.35072042915,18.1888571775611,0.));
#82812=CARTESIAN_POINT('Ctrl Pts',(213.866148574452,17.2380446619407,0.));
#82813=CARTESIAN_POINT('Ctrl Pts',(213.866148574452,17.2380446619407,17.2380446619407));
#82814=CARTESIAN_POINT('Ctrl Pts',(213.866148574452,0.,17.2380446619407));
#82815=CARTESIAN_POINT('Ctrl Pts',(213.866148574452,-17.2380446619407,17.2380446619407));
#82816=CARTESIAN_POINT('Ctrl Pts',(213.866148574452,-17.2380446619407,0.));
#82817=CARTESIAN_POINT('Ctrl Pts',(213.866148574452,-17.2380446619407,-17.2380446619407));
#82818=CARTESIAN_POINT('Ctrl Pts',(213.866148574452,0.,-17.2380446619407));
#82819=CARTESIAN_POINT('Ctrl Pts',(213.866148574452,17.2380446619407,-17.2380446619407));
#82820=CARTESIAN_POINT('Ctrl Pts',(213.866148574452,17.2380446619407,0.));
#82821=CARTESIAN_POINT('Ctrl Pts',(214.359054583237,16.3478426577189,0.));
#82822=CARTESIAN_POINT('Ctrl Pts',(214.359054583237,16.3478426577189,16.3478426577189));
#82823=CARTESIAN_POINT('Ctrl Pts',(214.359054583237,0.,16.3478426577189));
#82824=CARTESIAN_POINT('Ctrl Pts',(214.359054583237,-16.3478426577189,16.3478426577189));
#82825=CARTESIAN_POINT('Ctrl Pts',(214.359054583237,-16.3478426577189,0.));
#82826=CARTESIAN_POINT('Ctrl Pts',(214.359054583237,-16.3478426577189,-16.3478426577189));
#82827=CARTESIAN_POINT('Ctrl Pts',(214.359054583237,0.,-16.3478426577189));
#82828=CARTESIAN_POINT('Ctrl Pts',(214.359054583237,16.3478426577189,-16.3478426577189));
#82829=CARTESIAN_POINT('Ctrl Pts',(214.359054583237,16.3478426577189,0.));
#82830=CARTESIAN_POINT('Ctrl Pts',(214.822758777503,15.5577141109337,0.));
#82831=CARTESIAN_POINT('Ctrl Pts',(214.822758777503,15.5577141109337,15.5577141109337));
#82832=CARTESIAN_POINT('Ctrl Pts',(214.822758777503,0.,15.5577141109337));
#82833=CARTESIAN_POINT('Ctrl Pts',(214.822758777503,-15.5577141109337,15.5577141109337));
#82834=CARTESIAN_POINT('Ctrl Pts',(214.822758777503,-15.5577141109337,0.));
#82835=CARTESIAN_POINT('Ctrl Pts',(214.822758777503,-15.5577141109337,-15.5577141109337));
#82836=CARTESIAN_POINT('Ctrl Pts',(214.822758777503,0.,-15.5577141109337));
#82837=CARTESIAN_POINT('Ctrl Pts',(214.822758777503,15.5577141109337,-15.5577141109337));
#82838=CARTESIAN_POINT('Ctrl Pts',(214.822758777503,15.5577141109337,0.));
#82839=CARTESIAN_POINT('Ctrl Pts',(215.253384711971,14.8908052413081,0.));
#82840=CARTESIAN_POINT('Ctrl Pts',(215.253384711971,14.8908052413081,14.8908052413081));
#82841=CARTESIAN_POINT('Ctrl Pts',(215.253384711971,0.,14.8908052413081));
#82842=CARTESIAN_POINT('Ctrl Pts',(215.253384711971,-14.8908052413081,14.8908052413081));
#82843=CARTESIAN_POINT('Ctrl Pts',(215.253384711971,-14.8908052413081,0.));
#82844=CARTESIAN_POINT('Ctrl Pts',(215.253384711971,-14.8908052413081,-14.8908052413081));
#82845=CARTESIAN_POINT('Ctrl Pts',(215.253384711971,0.,-14.8908052413081));
#82846=CARTESIAN_POINT('Ctrl Pts',(215.253384711971,14.8908052413081,-14.8908052413081));
#82847=CARTESIAN_POINT('Ctrl Pts',(215.253384711971,14.8908052413081,0.));
#82848=CARTESIAN_POINT('Ctrl Pts',(215.569857199733,14.4651749705024,0.));
#82849=CARTESIAN_POINT('Ctrl Pts',(215.569857199733,14.4651749705024,14.4651749705024));
#82850=CARTESIAN_POINT('Ctrl Pts',(215.569857199733,0.,14.4651749705024));
#82851=CARTESIAN_POINT('Ctrl Pts',(215.569857199733,-14.4651749705024,14.4651749705024));
#82852=CARTESIAN_POINT('Ctrl Pts',(215.569857199733,-14.4651749705024,0.));
#82853=CARTESIAN_POINT('Ctrl Pts',(215.569857199733,-14.4651749705024,-14.4651749705024));
#82854=CARTESIAN_POINT('Ctrl Pts',(215.569857199733,0.,-14.4651749705024));
#82855=CARTESIAN_POINT('Ctrl Pts',(215.569857199733,14.4651749705024,-14.4651749705024));
#82856=CARTESIAN_POINT('Ctrl Pts',(215.569857199733,14.4651749705024,0.));
#82857=CARTESIAN_POINT('Ctrl Pts',(215.791167183037,14.2083320602137,0.));
#82858=CARTESIAN_POINT('Ctrl Pts',(215.791167183037,14.2083320602137,14.2083320602137));
#82859=CARTESIAN_POINT('Ctrl Pts',(215.791167183037,0.,14.2083320602137));
#82860=CARTESIAN_POINT('Ctrl Pts',(215.791167183037,-14.2083320602137,14.2083320602137));
#82861=CARTESIAN_POINT('Ctrl Pts',(215.791167183037,-14.2083320602137,0.));
#82862=CARTESIAN_POINT('Ctrl Pts',(215.791167183037,-14.2083320602137,-14.2083320602137));
#82863=CARTESIAN_POINT('Ctrl Pts',(215.791167183037,0.,-14.2083320602137));
#82864=CARTESIAN_POINT('Ctrl Pts',(215.791167183037,14.2083320602137,-14.2083320602137));
#82865=CARTESIAN_POINT('Ctrl Pts',(215.791167183037,14.2083320602137,0.));
#82866=CARTESIAN_POINT('Ctrl Pts',(215.931577335762,14.0648240477239,0.));
#82867=CARTESIAN_POINT('Ctrl Pts',(215.931577335762,14.0648240477239,14.0648240477239));
#82868=CARTESIAN_POINT('Ctrl Pts',(215.931577335762,0.,14.0648240477239));
#82869=CARTESIAN_POINT('Ctrl Pts',(215.931577335762,-14.0648240477239,14.0648240477239));
#82870=CARTESIAN_POINT('Ctrl Pts',(215.931577335762,-14.0648240477239,0.));
#82871=CARTESIAN_POINT('Ctrl Pts',(215.931577335762,-14.0648240477239,-14.0648240477239));
#82872=CARTESIAN_POINT('Ctrl Pts',(215.931577335762,0.,-14.0648240477239));
#82873=CARTESIAN_POINT('Ctrl Pts',(215.931577335762,14.0648240477239,-14.0648240477239));
#82874=CARTESIAN_POINT('Ctrl Pts',(215.931577335762,14.0648240477239,0.));
#82875=CARTESIAN_POINT('Ctrl Pts',(216.,14.,0.));
#82876=CARTESIAN_POINT('Ctrl Pts',(216.,14.,14.));
#82877=CARTESIAN_POINT('Ctrl Pts',(216.,0.,14.));
#82878=CARTESIAN_POINT('Ctrl Pts',(216.,-14.,14.));
#82879=CARTESIAN_POINT('Ctrl Pts',(216.,-14.,0.));
#82880=CARTESIAN_POINT('Ctrl Pts',(216.,-14.,-14.));
#82881=CARTESIAN_POINT('Ctrl Pts',(216.,0.,-14.));
#82882=CARTESIAN_POINT('Ctrl Pts',(216.,14.,-14.));
#82883=CARTESIAN_POINT('Ctrl Pts',(216.,14.,0.));
#82884=CARTESIAN_POINT('',(166.5,38.5,0.));
#82885=CARTESIAN_POINT('Ctrl Pts',(216.,14.,0.));
#82886=CARTESIAN_POINT('Ctrl Pts',(215.931577335762,14.0648240477239,0.));
#82887=CARTESIAN_POINT('Ctrl Pts',(215.791167183037,14.2083320602137,0.));
#82888=CARTESIAN_POINT('Ctrl Pts',(215.569857199733,14.4651749705024,0.));
#82889=CARTESIAN_POINT('Ctrl Pts',(215.253384711971,14.8908052413081,0.));
#82890=CARTESIAN_POINT('Ctrl Pts',(214.822758777503,15.5577141109337,0.));
#82891=CARTESIAN_POINT('Ctrl Pts',(214.359054583237,16.3478426577189,0.));
#82892=CARTESIAN_POINT('Ctrl Pts',(213.866148574452,17.2380446619407,0.));
#82893=CARTESIAN_POINT('Ctrl Pts',(213.35072042915,18.1888571775611,0.));
#82894=CARTESIAN_POINT('Ctrl Pts',(212.822218578073,19.1433606114324,0.));
#82895=CARTESIAN_POINT('Ctrl Pts',(212.290210763329,20.0360509959614,0.));
#82896=CARTESIAN_POINT('Ctrl Pts',(211.762347225289,20.7998079091476,0.));
#82897=CARTESIAN_POINT('Ctrl Pts',(211.241810802359,21.3737042041621,0.));
#82898=CARTESIAN_POINT('Ctrl Pts',(210.725601433264,21.7102505096364,0.));
#82899=CARTESIAN_POINT('Ctrl Pts',(210.200918116375,21.7834157131811,0.));
#82900=CARTESIAN_POINT('Ctrl Pts',(209.648738296528,21.5942508361551,0.));
#82901=CARTESIAN_POINT('Ctrl Pts',(209.053888810014,21.1748081323919,0.));
#82902=CARTESIAN_POINT('Ctrl Pts',(208.412972675131,20.5920992378761,0.));
#82903=CARTESIAN_POINT('Ctrl Pts',(207.744015652215,19.9532689458847,0.));
#82904=CARTESIAN_POINT('Ctrl Pts',(207.078090239928,19.3848418671143,0.));
#82905=CARTESIAN_POINT('Ctrl Pts',(206.449692896782,19.0096950757953,0.));
#82906=CARTESIAN_POINT('Ctrl Pts',(205.887941237232,18.9257935294742,0.));
#82907=CARTESIAN_POINT('Ctrl Pts',(205.406561032152,19.1819945300443,0.));
#82908=CARTESIAN_POINT('Ctrl Pts',(204.996948764239,19.7615251622739,0.));
#82909=CARTESIAN_POINT('Ctrl Pts',(204.636303489551,20.6033665580493,0.));
#82910=CARTESIAN_POINT('Ctrl Pts',(204.293916519169,21.6189881673319,0.));
#82911=CARTESIAN_POINT('Ctrl Pts',(203.937951189067,22.7103152246357,0.));
#82912=CARTESIAN_POINT('Ctrl Pts',(203.542511863345,23.7884093162236,0.));
#82913=CARTESIAN_POINT('Ctrl Pts',(203.093076162889,24.7880448411392,0.));
#82914=CARTESIAN_POINT('Ctrl Pts',(202.583897300149,25.6620387985065,0.));
#82915=CARTESIAN_POINT('Ctrl Pts',(202.016556766229,26.3785672681198,0.));
#82916=CARTESIAN_POINT('Ctrl Pts',(201.39806187553,26.9171117141031,0.));
#82917=CARTESIAN_POINT('Ctrl Pts',(200.739177478596,27.2655121051523,0.));
#82918=CARTESIAN_POINT('Ctrl Pts',(200.052580368893,27.4153142520686,0.));
#82919=CARTESIAN_POINT('Ctrl Pts',(199.351380905309,27.3622787234429,0.));
#82920=CARTESIAN_POINT('Ctrl Pts',(198.64812240998,27.1147192657497,0.));
#82921=CARTESIAN_POINT('Ctrl Pts',(197.953680886587,26.6997761508392,0.));
#82922=CARTESIAN_POINT('Ctrl Pts',(197.27617886607,26.1710294150248,0.));
#82923=CARTESIAN_POINT('Ctrl Pts',(196.61996014565,25.6142225395129,0.));
#82924=CARTESIAN_POINT('Ctrl Pts',(195.986035381944,25.1290290983464,0.));
#82925=CARTESIAN_POINT('Ctrl Pts',(195.372421781966,24.8112917102097,0.));
#82926=CARTESIAN_POINT('Ctrl Pts',(194.774568374152,24.7365253484543,0.));
#82927=CARTESIAN_POINT('Ctrl Pts',(194.185626322862,24.9394496497274,0.));
#82928=CARTESIAN_POINT('Ctrl Pts',(193.597176293606,25.4069487182106,0.));
#82929=CARTESIAN_POINT('Ctrl Pts',(193.000672363666,26.0939712858825,0.));
#82930=CARTESIAN_POINT('Ctrl Pts',(192.388791155139,26.9344733292055,0.));
#82931=CARTESIAN_POINT('Ctrl Pts',(191.756675094258,27.853709335318,0.));
#82932=CARTESIAN_POINT('Ctrl Pts',(191.103572014169,28.781420151568,0.));
#82933=CARTESIAN_POINT('Ctrl Pts',(190.433084076035,29.6594255092613,0.));
#82934=CARTESIAN_POINT('Ctrl Pts',(189.75112407993,30.4394160167154,0.));
#82935=CARTESIAN_POINT('Ctrl Pts',(189.064450793941,31.0831127500011,0.));
#82936=CARTESIAN_POINT('Ctrl Pts',(188.37888266216,31.5613864248805,0.));
#82937=CARTESIAN_POINT('Ctrl Pts',(187.697855441439,31.854052831669,0.));
#82938=CARTESIAN_POINT('Ctrl Pts',(187.020322757229,31.9488468045685,0.));
#82939=CARTESIAN_POINT('Ctrl Pts',(186.340814647256,31.8427771137434,0.));
#82940=CARTESIAN_POINT('Ctrl Pts',(185.652242796566,31.546505030526,0.));
#82941=CARTESIAN_POINT('Ctrl Pts',(184.947972925117,31.0878161213455,0.));
#82942=CARTESIAN_POINT('Ctrl Pts',(184.224280732459,30.5158363027008,0.));
#82943=CARTESIAN_POINT('Ctrl Pts',(183.482400836276,29.9039282850736,0.));
#82944=CARTESIAN_POINT('Ctrl Pts',(182.726909789558,29.3367202018516,0.));
#82945=CARTESIAN_POINT('Ctrl Pts',(181.964356356054,28.8984085343652,0.));
#82946=CARTESIAN_POINT('Ctrl Pts',(181.201754230035,28.660085613321,0.));
#82947=CARTESIAN_POINT('Ctrl Pts',(180.445242944925,28.6686083897625,0.));
#82948=CARTESIAN_POINT('Ctrl Pts',(179.69839696542,28.9318633546098,0.));
#82949=CARTESIAN_POINT('Ctrl Pts',(178.962404276569,29.4235353639997,0.));
#82950=CARTESIAN_POINT('Ctrl Pts',(178.236882848697,30.0945584620795,0.));
#82951=CARTESIAN_POINT('Ctrl Pts',(177.520501166053,30.8825005559741,0.));
#82952=CARTESIAN_POINT('Ctrl Pts',(176.811644553588,31.7214384106704,0.));
#82953=CARTESIAN_POINT('Ctrl Pts',(176.10914445329,32.5524621154421,0.));
#82954=CARTESIAN_POINT('Ctrl Pts',(175.412716697241,33.3312296578559,0.));
#82955=CARTESIAN_POINT('Ctrl Pts',(174.722485008373,34.0263777716625,0.));
#82956=CARTESIAN_POINT('Ctrl Pts',(174.038678741555,34.6195419357237,0.));
#82957=CARTESIAN_POINT('Ctrl Pts',(173.361242516346,35.1048554959833,0.));
#82958=CARTESIAN_POINT('Ctrl Pts',(172.689527753591,35.4884519662692,0.));
#82959=CARTESIAN_POINT('Ctrl Pts',(172.021839116729,35.7885524264098,0.));
#82960=CARTESIAN_POINT('Ctrl Pts',(171.355454837575,36.0331538549227,0.));
#82961=CARTESIAN_POINT('Ctrl Pts',(170.687195598755,36.25481814225,0.));
#82962=CARTESIAN_POINT('Ctrl Pts',(170.013852859503,36.4862057554389,0.));
#82963=CARTESIAN_POINT('Ctrl Pts',(169.332671034328,36.7553393532152,0.));
#82964=CARTESIAN_POINT('Ctrl Pts',(168.641815524474,37.0808938108885,0.));
#82965=CARTESIAN_POINT('Ctrl Pts',(167.940195292269,37.4740045272214,0.));
#82966=CARTESIAN_POINT('Ctrl Pts',(167.369855715636,37.8469615594215,0.));
#82967=CARTESIAN_POINT('Ctrl Pts',(166.936935989037,38.1603786909402,0.));
#82968=CARTESIAN_POINT('Ctrl Pts',(166.646027830324,38.384297265584,0.));
#82969=CARTESIAN_POINT('Ctrl Pts',(166.5,38.5,0.));
#82970=CARTESIAN_POINT('',(166.5,-38.5,-4.71489017671731E-15));
#82971=CARTESIAN_POINT('Origin',(166.5,0.,0.));
#82972=CARTESIAN_POINT('Origin',(166.5,0.,0.));
#82973=CARTESIAN_POINT('Origin',(166.25,0.,0.));
#82974=CARTESIAN_POINT('',(166.25,-39.25,-4.80673868665336E-15));
#90344=UNCERTAINTY_MEASURE_WITH_UNIT(LENGTH_MEASURE(0.01),#90375,
'DISTANCE_ACCURACY_VALUE',
'Maximum model space distance between geometric entities at asserted c
onnectivities');
#90355=UNCERTAINTY_MEASURE_WITH_UNIT(LENGTH_MEASURE(0.01),#90375,
'DISTANCE_ACCURACY_VALUE',
'Maximum model space distance between geometric entities at asserted c
onnectivities');
#90363=(
GEOMETRIC_REPRESENTATION_CONTEXT(3)
GLOBAL_UNCERTAINTY_ASSIGNED_CONTEXT((#90344))
GLOBAL_UNIT_ASSIGNED_CONTEXT((#90375,#90377,#90378))
REPRESENTATION_CONTEXT('','3D')
);
#90374=(
GEOMETRIC_REPRESENTATION_CONTEXT(3)
GLOBAL_UNCERTAINTY_ASSIGNED_CONTEXT((#90355))
GLOBAL_UNIT_ASSIGNED_CONTEXT((#90375,#90377,#90378))
REPRESENTATION_CONTEXT('','3D')
);
#90375=(
LENGTH_UNIT()
NAMED_UNIT(*)
SI_UNIT(.MILLI.,.METRE.)
);
#90377=(
NAMED_UNIT(*)
PLANE_ANGLE_UNIT()
SI_UNIT($,.RADIAN.)
);
#90378=(
NAMED_UNIT(*)
SI_UNIT($,.STERADIAN.)
SOLID_ANGLE_UNIT()
);
#90386=SHAPE_DEFINITION_REPRESENTATION(#90404,#90447);
#90404=PRODUCT_DEFINITION_SHAPE('',$,#90466);
#90447=SHAPE_REPRESENTATION('',(#43795),#90363);
#90458=PRODUCT_DEFINITION_CONTEXT('part definition',#90514,'design');
#90466=PRODUCT_DEFINITION('2026-10-11-12-53-10-690','07_Outer_CV_Boot',
#90484,#90458);
#90484=PRODUCT_DEFINITION_FORMATION('',$,#90523);
#90514=APPLICATION_CONTEXT(
'Core Data for Automotive Mechanical Design Process');
#90515=PRODUCT_CONTEXT('part definition',#90514,'mechanical');
#90523=PRODUCT('2026-10-11-12-53-10-690','07_Outer_CV_Boot',$,(#90515));
#90674=COLOUR_RGB('Sky Blue',0.24,0.69,0.87);
#90675=FILL_AREA_STYLE_COLOUR('',#90674);
#90676=FILL_AREA_STYLE('',(#90675));
#90677=SURFACE_STYLE_FILL_AREA(#90676);
#90678=SURFACE_SIDE_STYLE('',(#90677));
#90679=SURFACE_STYLE_USAGE(.BOTH.,#90678);
#90680=PRESENTATION_STYLE_ASSIGNMENT((#90679));
ENDSEC;
END-ISO-10303-21;
